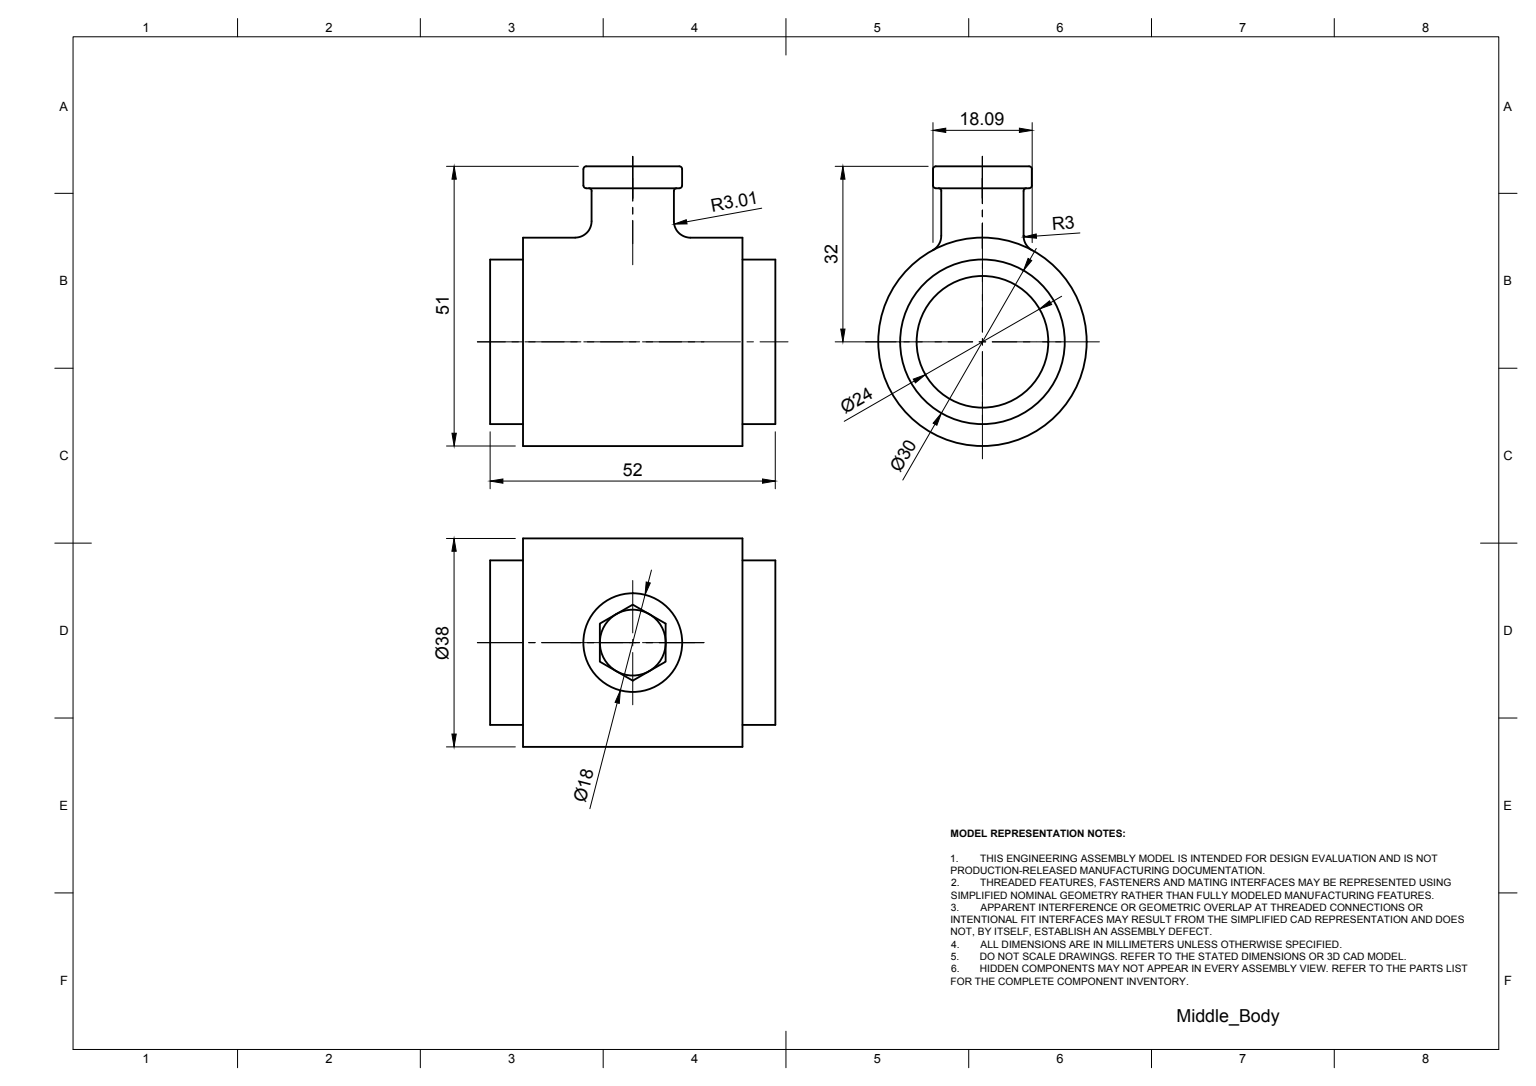
ISO-10303-21;
HEADER;
/* Generated by software containing ST-Developer
 * from STEP Tools, Inc. (www.steptools.com) 
 */

FILE_DESCRIPTION(
/* description */ (''),
/* implementation_level */ '2;1');

FILE_NAME(
/* name */ 'Middle_Body.step',
/* time_stamp */ '2026-10-06T12:47:13-07:00',
/* author */ (''),
/* organization */ (''),
/* preprocessor_version */ 'ST-DEVELOPER v20.2',
/* originating_system */ 'Autodesk Translation Framework v15.15.0.0',
/* authorisation */ '');

FILE_SCHEMA (('AUTOMOTIVE_DESIGN { 1 0 10303 214 3 1 1 }'));
ENDSEC;

DATA;
#10=MECHANICAL_DESIGN_GEOMETRIC_PRESENTATION_REPRESENTATION('',(#67),#42667);
#49=SHAPE_REPRESENTATION_RELATIONSHIP('SRR','None',#42702,#58);
#58=ADVANCED_BREP_SHAPE_REPRESENTATION('',(#76),#42658);
#67=STYLED_ITEM('',(#42756),#76);
#76=MANIFOLD_SOLID_BREP('Body1',#4032);
#85=B_SPLINE_SURFACE_WITH_KNOTS('',3,3,((#5678,#5679,#5680,#5681,#5682,
#5683,#5684,#5685,#5686,#5687,#5688,#5689,#5690,#5691,#5692,#5693,#5694,
#5695),(#5696,#5697,#5698,#5699,#5700,#5701,#5702,#5703,#5704,#5705,#5706,
#5707,#5708,#5709,#5710,#5711,#5712,#5713),(#5714,#5715,#5716,#5717,#5718,
#5719,#5720,#5721,#5722,#5723,#5724,#5725,#5726,#5727,#5728,#5729,#5730,
#5731),(#5732,#5733,#5734,#5735,#5736,#5737,#5738,#5739,#5740,#5741,#5742,
#5743,#5744,#5745,#5746,#5747,#5748,#5749),(#5750,#5751,#5752,#5753,#5754,
#5755,#5756,#5757,#5758,#5759,#5760,#5761,#5762,#5763,#5764,#5765,#5766,
#5767)),.UNSPECIFIED.,.F.,.T.,.F.,(4,1,4),(4,1,1,1,1,1,1,1,1,1,1,1,1,1,
1,4),(0.,0.571428571428571,1.00004196138552),(0.,0.326770108848208,0.653540217696416,
0.980310326544624,1.30708043539283,1.52492717462497,1.96062065308925,2.17846739232139,
2.39631413155352,2.61416087078566,3.04985434924994,3.26770108848208,3.48554782771422,
3.92124130617849,4.2480114150267,4.57478152387491),.UNSPECIFIED.);
#94=B_SPLINE_CURVE_WITH_KNOTS('',3,(#5427,#5428,#5429,#5430,#5431,#5432,
#5433,#5434,#5435,#5436,#5437,#5438,#5439,#5440,#5441,#5442,#5443,#5444,
#5445,#5446,#5447,#5448,#5449,#5450,#5451,#5452,#5453,#5454,#5455,#5456,
#5457,#5458,#5459,#5460,#5461,#5462,#5463,#5464,#5465,#5466,#5467,#5468,
#5469,#5470,#5471,#5472,#5473,#5474,#5475,#5476,#5477,#5478,#5479,#5480,
#5481,#5482,#5483,#5484,#5485,#5486,#5487,#5488,#5489,#5490,#5491,#5492,
#5493,#5494,#5495,#5496,#5497,#5498,#5499,#5500,#5501,#5502,#5503,#5504,
#5505,#5506,#5507,#5508,#5509,#5510,#5511,#5512,#5513,#5514,#5515,#5516,
#5517,#5518,#5519,#5520,#5521,#5522,#5523,#5524,#5525,#5526,#5527,#5528,
#5529,#5530,#5531,#5532,#5533,#5534,#5535,#5536,#5537,#5538,#5539,#5540,
#5541,#5542,#5543,#5544,#5545,#5546,#5547,#5548,#5549,#5550),
 .UNSPECIFIED.,.F.,.F.,(4,3,3,3,3,3,3,3,3,3,3,3,3,3,3,3,3,3,3,3,3,3,3,3,
3,3,3,3,3,3,3,3,3,3,3,3,3,3,3,3,3,4),(0.,0.0515890274929282,0.103204292695659,
0.154856373216778,0.206591856648151,0.25837614825577,0.310254566416546,
0.326770108848208,0.398899776939704,0.480730369472977,0.567135293584696,
0.646990791668246,0.653540217696416,0.713270639311335,0.772778129234328,
0.831949962874738,0.890922354735589,0.949595703830974,0.980310326544624,
1.02811421917601,1.07588590458137,1.1236371825647,1.17139353825776,1.21915060551796,
1.26694469505578,1.30708043539283,1.36339088247901,1.4198291936612,1.47649599617247,
1.52492717462497,1.60478198943241,1.69630632876662,1.79926962978145,1.88030337649094,
1.96062065308925,2.01516322116673,2.0696000908893,2.12403374160535,2.17846739232139,
2.22502234109762,2.27155796869371,2.28737840760206),.UNSPECIFIED.);
#95=B_SPLINE_CURVE_WITH_KNOTS('',3,(#5551,#5552,#5553,#5554,#5555,#5556,
#5557,#5558,#5559,#5560,#5561,#5562,#5563,#5564,#5565,#5566,#5567,#5568,
#5569,#5570,#5571,#5572,#5573,#5574,#5575,#5576,#5577,#5578,#5579,#5580,
#5581,#5582,#5583,#5584,#5585,#5586,#5587,#5588,#5589,#5590,#5591,#5592,
#5593,#5594,#5595,#5596,#5597,#5598,#5599,#5600,#5601,#5602,#5603,#5604,
#5605,#5606,#5607,#5608,#5609,#5610,#5611,#5612,#5613,#5614,#5615,#5616,
#5617,#5618,#5619,#5620,#5621,#5622,#5623,#5624,#5625,#5626,#5627,#5628,
#5629,#5630,#5631,#5632,#5633,#5634,#5635,#5636,#5637,#5638,#5639,#5640,
#5641,#5642,#5643,#5644,#5645,#5646,#5647,#5648,#5649,#5650,#5651,#5652,
#5653,#5654,#5655,#5656,#5657,#5658,#5659,#5660,#5661,#5662,#5663,#5664,
#5665,#5666,#5667,#5668,#5669,#5670,#5671,#5672,#5673,#5674,#5675,#5676,
#5677),.UNSPECIFIED.,.F.,.F.,(4,3,3,3,3,3,3,3,3,3,3,3,3,3,3,3,3,3,3,3,3,
3,3,3,3,3,3,3,3,3,3,3,3,3,3,3,3,3,3,3,3,3,4),(2.28737840766402,2.33375007519743,
2.3801437049756,2.39631413155352,2.45117314344955,2.50612653591306,2.56126498980737,
2.61416087078566,2.69133411582037,2.77539876579215,2.86930017643718,2.95957726284356,
3.0384899988861,3.04985434924994,3.11071114418125,3.17119439820841,3.23109353713712,
3.26770108848208,3.31260298810012,3.35748093451019,3.40234653816875,3.44723256342706,
3.48554782771422,3.54204675587125,3.59866131344456,3.65539681169898,3.712258631246,
3.76933145073308,3.82652040574213,3.8839071682845,3.92124130617849,4.00407786973751,
4.08802290404028,4.16801715953349,4.23929616483205,4.2480114150267,4.30052474757075,
4.35295604051741,4.40531606758536,4.45759990073163,4.50983970731316,4.56203893311869,
4.57478152387491),.UNSPECIFIED.);
#96=B_SPLINE_CURVE_WITH_KNOTS('',3,(#5769,#5770,#5771,#5772,#5773),
 .UNSPECIFIED.,.F.,.F.,(4,1,4),(0.,0.571428571428571,1.00000000000031),
 .UNSPECIFIED.);
#97=B_SPLINE_CURVE_WITH_KNOTS('',3,(#5774,#5775,#5776,#5777,#5778,#5779,
#5780,#5781,#5782,#5783,#5784,#5785,#5786,#5787,#5788,#5789,#5790,#5791),
 .UNSPECIFIED.,.T.,.F.,(4,1,1,1,1,1,1,1,1,1,1,1,1,1,1,4),(-4.57478152387491,
-4.2480114150267,-3.92124130617849,-3.48554782771422,-3.26770108848208,
-3.04985434924994,-2.61416087078566,-2.39631413155352,-2.17846739232139,
-1.96062065308925,-1.52492717462497,-1.30708043539283,-0.980310326544624,
-0.653540217696416,-0.326770108848208,0.),.UNSPECIFIED.);
#98=B_SPLINE_CURVE_WITH_KNOTS('',3,(#5801,#5802,#5803,#5804,#5805,#5806,
#5807,#5808,#5809,#5810,#5811,#5812,#5813,#5814,#5815,#5816,#5817,#5818),
 .UNSPECIFIED.,.F.,.F.,(4,2,2,2,2,2,2,2,4),(-3.69014930019619,-3.45920017966731,
-3.22825105913842,-2.99793151714278,-2.76761197514714,-2.5372924331515,
-2.30697289115586,-2.07602377062698,-1.8450746500981),.UNSPECIFIED.);
#99=B_SPLINE_CURVE_WITH_KNOTS('',3,(#5819,#5820,#5821,#5822,#5823,#5824,
#5825,#5826,#5827,#5828,#5829,#5830,#5831,#5832,#5833,#5834,#5835,#5836),
 .UNSPECIFIED.,.F.,.F.,(4,2,2,2,2,2,2,2,4),(-1.8450746500981,-1.61412552956921,
-1.38317640904033,-1.15285686704469,-0.922537325049048,-0.692217783053408,
-0.461898241057768,-0.230949120528884,0.),.UNSPECIFIED.);
#379=FACE_BOUND('',#851,.T.);
#380=FACE_BOUND('',#854,.T.);
#381=FACE_BOUND('',#859,.T.);
#382=FACE_BOUND('',#863,.T.);
#383=FACE_BOUND('',#866,.T.);
#384=FACE_BOUND('',#868,.T.);
#385=FACE_BOUND('',#870,.T.);
#386=FACE_BOUND('',#872,.T.);
#396=CYLINDRICAL_SURFACE('',#4166,9.);
#397=CYLINDRICAL_SURFACE('',#4178,7.5);
#398=CYLINDRICAL_SURFACE('',#4179,19.);
#399=CYLINDRICAL_SURFACE('',#4182,6.);
#400=CYLINDRICAL_SURFACE('',#4183,15.);
#401=CYLINDRICAL_SURFACE('',#4188,15.);
#402=CYLINDRICAL_SURFACE('',#4193,12.);
#500=TOROIDAL_SURFACE('',#4162,8.5,0.5);
#501=TOROIDAL_SURFACE('',#4169,8.5,0.5);
#502=TOROIDAL_SURFACE('',#4174,8.,0.5);
#519=CIRCLE('',#4148,6.);
#520=CIRCLE('',#4150,6.);
#521=CIRCLE('',#4152,6.);
#522=CIRCLE('',#4154,6.);
#523=CIRCLE('',#4156,6.);
#524=CIRCLE('',#4158,6.);
#525=CIRCLE('',#4159,6.);
#526=CIRCLE('',#4163,8.5);
#527=CIRCLE('',#4164,0.5);
#528=CIRCLE('',#4165,9.);
#529=CIRCLE('',#4167,9.);
#530=CIRCLE('',#4170,0.5);
#531=CIRCLE('',#4171,8.5);
#532=CIRCLE('',#4173,8.);
#533=CIRCLE('',#4175,7.5);
#534=CIRCLE('',#4176,0.5);
#535=CIRCLE('',#4177,7.5);
#536=CIRCLE('',#4180,19.);
#537=CIRCLE('',#4181,19.);
#538=CIRCLE('',#4184,15.);
#539=CIRCLE('',#4185,15.);
#540=CIRCLE('',#4187,12.);
#541=CIRCLE('',#4189,15.);
#542=CIRCLE('',#4190,15.);
#543=CIRCLE('',#4192,12.);
#638=FACE_OUTER_BOUND('',#836,.T.);
#639=FACE_OUTER_BOUND('',#837,.T.);
#640=FACE_OUTER_BOUND('',#838,.T.);
#641=FACE_OUTER_BOUND('',#839,.T.);
#642=FACE_OUTER_BOUND('',#840,.T.);
#643=FACE_OUTER_BOUND('',#841,.T.);
#644=FACE_OUTER_BOUND('',#842,.T.);
#645=FACE_OUTER_BOUND('',#843,.T.);
#646=FACE_OUTER_BOUND('',#844,.T.);
#647=FACE_OUTER_BOUND('',#845,.T.);
#648=FACE_OUTER_BOUND('',#846,.T.);
#649=FACE_OUTER_BOUND('',#847,.T.);
#650=FACE_OUTER_BOUND('',#848,.T.);
#651=FACE_OUTER_BOUND('',#849,.T.);
#652=FACE_OUTER_BOUND('',#850,.T.);
#653=FACE_OUTER_BOUND('',#852,.T.);
#654=FACE_OUTER_BOUND('',#853,.T.);
#655=FACE_OUTER_BOUND('',#855,.T.);
#656=FACE_OUTER_BOUND('',#856,.T.);
#657=FACE_OUTER_BOUND('',#857,.T.);
#658=FACE_OUTER_BOUND('',#858,.T.);
#659=FACE_OUTER_BOUND('',#860,.T.);
#660=FACE_OUTER_BOUND('',#861,.T.);
#661=FACE_OUTER_BOUND('',#862,.T.);
#662=FACE_OUTER_BOUND('',#864,.T.);
#663=FACE_OUTER_BOUND('',#865,.T.);
#664=FACE_OUTER_BOUND('',#867,.T.);
#665=FACE_OUTER_BOUND('',#869,.T.);
#666=FACE_OUTER_BOUND('',#871,.T.);
#836=EDGE_LOOP('',(#2536,#2537,#2538,#2539,#2540));
#837=EDGE_LOOP('',(#2541,#2542,#2543,#2544,#2545));
#838=EDGE_LOOP('',(#2546,#2547,#2548,#2549,#2550));
#839=EDGE_LOOP('',(#2551,#2552,#2553,#2554,#2555));
#840=EDGE_LOOP('',(#2556,#2557,#2558));
#841=EDGE_LOOP('',(#2559,#2560,#2561));
#842=EDGE_LOOP('',(#2562,#2563,#2564));
#843=EDGE_LOOP('',(#2565,#2566,#2567));
#844=EDGE_LOOP('',(#2568,#2569,#2570));
#845=EDGE_LOOP('',(#2571,#2572,#2573,#2574));
#846=EDGE_LOOP('',(#2575,#2576,#2577,#2578,#2579));
#847=EDGE_LOOP('',(#2580,#2581,#2582,#2583,#2584));
#848=EDGE_LOOP('',(#2585,#2586,#2587,#2588));
#849=EDGE_LOOP('',(#2589,#2590,#2591,#2592));
#850=EDGE_LOOP('',(#2593));
#851=EDGE_LOOP('',(#2594,#2595,#2596,#2597,#2598,#2599));
#852=EDGE_LOOP('',(#2600,#2601,#2602,#2603));
#853=EDGE_LOOP('',(#2604));
#854=EDGE_LOOP('',(#2605));
#855=EDGE_LOOP('',(#2606,#2607,#2608,#2609,#2610));
#856=EDGE_LOOP('',(#2611,#2612,#2613,#2614,#2615,#2616));
#857=EDGE_LOOP('',(#2617,#2618,#2619,#2620,#2621));
#858=EDGE_LOOP('',(#2622,#2623,#2624,#2625));
#859=EDGE_LOOP('',(#2626));
#860=EDGE_LOOP('',(#2627,#2628,#2629,#2630,#2631,#2632,#2633,#2634,#2635,
#2636,#2637));
#861=EDGE_LOOP('',(#2638,#2639,#2640,#2641));
#862=EDGE_LOOP('',(#2642));
#863=EDGE_LOOP('',(#2643));
#864=EDGE_LOOP('',(#2644,#2645,#2646,#2647));
#865=EDGE_LOOP('',(#2648));
#866=EDGE_LOOP('',(#2649));
#867=EDGE_LOOP('',(#2650,#2651,#2652,#2653));
#868=EDGE_LOOP('',(#2654,#2655));
#869=EDGE_LOOP('',(#2656));
#870=EDGE_LOOP('',(#2657));
#871=EDGE_LOOP('',(#2658));
#872=EDGE_LOOP('',(#2659));
#1051=LINE('',#5340,#1264);
#1052=LINE('',#5342,#1265);
#1053=LINE('',#5344,#1266);
#1054=LINE('',#5346,#1267);
#1055=LINE('',#5347,#1268);
#1056=LINE('',#5350,#1269);
#1057=LINE('',#5352,#1270);
#1058=LINE('',#5354,#1271);
#1059=LINE('',#5355,#1272);
#1060=LINE('',#5358,#1273);
#1061=LINE('',#5360,#1274);
#1062=LINE('',#5362,#1275);
#1063=LINE('',#5363,#1276);
#1064=LINE('',#5366,#1277);
#1065=LINE('',#5368,#1278);
#1066=LINE('',#5370,#1279);
#1067=LINE('',#5371,#1280);
#1068=LINE('',#5377,#1281);
#1069=LINE('',#5378,#1282);
#1070=LINE('',#5381,#1283);
#1071=LINE('',#5391,#1284);
#1072=LINE('',#5395,#1285);
#1073=LINE('',#5396,#1286);
#1074=LINE('',#5398,#1287);
#1075=LINE('',#5407,#1288);
#1076=LINE('',#5425,#1289);
#1077=LINE('',#5796,#1290);
#1078=LINE('',#5837,#1291);
#1079=LINE('',#5842,#1292);
#1080=LINE('',#5851,#1293);
#1081=LINE('',#5857,#1294);
#1264=VECTOR('',#4474,10.);
#1265=VECTOR('',#4475,10.);
#1266=VECTOR('',#4476,10.);
#1267=VECTOR('',#4477,10.);
#1268=VECTOR('',#4478,10.);
#1269=VECTOR('',#4481,10.);
#1270=VECTOR('',#4482,10.);
#1271=VECTOR('',#4483,10.);
#1272=VECTOR('',#4484,10.);
#1273=VECTOR('',#4487,10.);
#1274=VECTOR('',#4488,10.);
#1275=VECTOR('',#4489,10.);
#1276=VECTOR('',#4490,10.);
#1277=VECTOR('',#4493,9.99999999999999);
#1278=VECTOR('',#4494,10.);
#1279=VECTOR('',#4495,9.99999999999999);
#1280=VECTOR('',#4496,9.99999999999999);
#1281=VECTOR('',#4501,10.);
#1282=VECTOR('',#4502,10.);
#1283=VECTOR('',#4507,10.);
#1284=VECTOR('',#4524,10.);
#1285=VECTOR('',#4529,10.);
#1286=VECTOR('',#4530,10.);
#1287=VECTOR('',#4533,10.);
#1288=VECTOR('',#4544,9.);
#1289=VECTOR('',#4569,7.5);
#1290=VECTOR('',#4574,19.);
#1291=VECTOR('',#4579,6.);
#1292=VECTOR('',#4584,15.);
#1293=VECTOR('',#4595,15.);
#1294=VECTOR('',#4604,12.);
#1477=VERTEX_POINT('',#5338);
#1478=VERTEX_POINT('',#5339);
#1479=VERTEX_POINT('',#5341);
#1480=VERTEX_POINT('',#5343);
#1481=VERTEX_POINT('',#5345);
#1482=VERTEX_POINT('',#5349);
#1483=VERTEX_POINT('',#5351);
#1484=VERTEX_POINT('',#5353);
#1485=VERTEX_POINT('',#5357);
#1486=VERTEX_POINT('',#5359);
#1487=VERTEX_POINT('',#5361);
#1488=VERTEX_POINT('',#5365);
#1489=VERTEX_POINT('',#5367);
#1490=VERTEX_POINT('',#5369);
#1491=VERTEX_POINT('',#5373);
#1492=VERTEX_POINT('',#5374);
#1493=VERTEX_POINT('',#5376);
#1494=VERTEX_POINT('',#5389);
#1495=VERTEX_POINT('',#5394);
#1496=VERTEX_POINT('',#5400);
#1497=VERTEX_POINT('',#5402);
#1498=VERTEX_POINT('',#5406);
#1499=VERTEX_POINT('',#5411);
#1500=VERTEX_POINT('',#5415);
#1501=VERTEX_POINT('',#5418);
#1502=VERTEX_POINT('',#5419);
#1503=VERTEX_POINT('',#5424);
#1504=VERTEX_POINT('',#5426);
#1505=VERTEX_POINT('',#5768);
#1506=VERTEX_POINT('',#5793);
#1507=VERTEX_POINT('',#5795);
#1508=VERTEX_POINT('',#5799);
#1509=VERTEX_POINT('',#5800);
#1510=VERTEX_POINT('',#5839);
#1511=VERTEX_POINT('',#5841);
#1512=VERTEX_POINT('',#5845);
#1513=VERTEX_POINT('',#5848);
#1514=VERTEX_POINT('',#5850);
#1515=VERTEX_POINT('',#5854);
#1919=EDGE_CURVE('',#1477,#1478,#1051,.T.);
#1920=EDGE_CURVE('',#1479,#1477,#1052,.T.);
#1921=EDGE_CURVE('',#1479,#1480,#1053,.T.);
#1922=EDGE_CURVE('',#1480,#1481,#1054,.T.);
#1923=EDGE_CURVE('',#1481,#1478,#1055,.T.);
#1924=EDGE_CURVE('',#1482,#1477,#1056,.T.);
#1925=EDGE_CURVE('',#1483,#1482,#1057,.T.);
#1926=EDGE_CURVE('',#1483,#1484,#1058,.T.);
#1927=EDGE_CURVE('',#1484,#1479,#1059,.T.);
#1928=EDGE_CURVE('',#1478,#1485,#1060,.T.);
#1929=EDGE_CURVE('',#1481,#1486,#1061,.T.);
#1930=EDGE_CURVE('',#1486,#1487,#1062,.T.);
#1931=EDGE_CURVE('',#1487,#1485,#1063,.T.);
#1932=EDGE_CURVE('',#1488,#1482,#1064,.T.);
#1933=EDGE_CURVE('',#1489,#1488,#1065,.T.);
#1934=EDGE_CURVE('',#1489,#1490,#1066,.T.);
#1935=EDGE_CURVE('',#1490,#1483,#1067,.T.);
#1936=EDGE_CURVE('',#1491,#1492,#519,.T.);
#1937=EDGE_CURVE('',#1493,#1491,#1068,.T.);
#1938=EDGE_CURVE('',#1492,#1493,#1069,.T.);
#1939=EDGE_CURVE('',#1492,#1486,#520,.T.);
#1940=EDGE_CURVE('',#1487,#1492,#1070,.T.);
#1941=EDGE_CURVE('',#1486,#1480,#521,.T.);
#1942=EDGE_CURVE('',#1480,#1484,#522,.T.);
#1943=EDGE_CURVE('',#1484,#1490,#523,.T.);
#1944=EDGE_CURVE('',#1490,#1494,#524,.T.);
#1945=EDGE_CURVE('',#1491,#1489,#1071,.T.);
#1946=EDGE_CURVE('',#1494,#1491,#525,.T.);
#1947=EDGE_CURVE('',#1485,#1495,#1072,.T.);
#1948=EDGE_CURVE('',#1495,#1493,#1073,.T.);
#1949=EDGE_CURVE('',#1495,#1488,#1074,.T.);
#1950=EDGE_CURVE('',#1496,#1496,#526,.T.);
#1951=EDGE_CURVE('',#1496,#1497,#527,.T.);
#1952=EDGE_CURVE('',#1497,#1497,#528,.T.);
#1953=EDGE_CURVE('',#1497,#1498,#1075,.T.);
#1954=EDGE_CURVE('',#1498,#1498,#529,.T.);
#1955=EDGE_CURVE('',#1498,#1499,#530,.T.);
#1956=EDGE_CURVE('',#1499,#1499,#531,.T.);
#1957=EDGE_CURVE('',#1500,#1500,#532,.T.);
#1958=EDGE_CURVE('',#1501,#1502,#533,.T.);
#1959=EDGE_CURVE('',#1502,#1500,#534,.T.);
#1960=EDGE_CURVE('',#1502,#1501,#535,.T.);
#1961=EDGE_CURVE('',#1501,#1503,#1076,.T.);
#1962=EDGE_CURVE('',#1504,#1503,#94,.T.);
#1963=EDGE_CURVE('',#1503,#1504,#95,.T.);
#1964=EDGE_CURVE('',#1505,#1504,#96,.T.);
#1965=EDGE_CURVE('',#1505,#1505,#97,.T.);
#1966=EDGE_CURVE('',#1506,#1506,#536,.T.);
#1967=EDGE_CURVE('',#1506,#1507,#1077,.T.);
#1968=EDGE_CURVE('',#1507,#1507,#537,.T.);
#1969=EDGE_CURVE('',#1508,#1509,#98,.T.);
#1970=EDGE_CURVE('',#1509,#1508,#99,.T.);
#1971=EDGE_CURVE('',#1509,#1494,#1078,.T.);
#1972=EDGE_CURVE('',#1510,#1510,#538,.T.);
#1973=EDGE_CURVE('',#1510,#1511,#1079,.T.);
#1974=EDGE_CURVE('',#1511,#1511,#539,.T.);
#1975=EDGE_CURVE('',#1512,#1512,#540,.T.);
#1976=EDGE_CURVE('',#1513,#1513,#541,.T.);
#1977=EDGE_CURVE('',#1513,#1514,#1080,.T.);
#1978=EDGE_CURVE('',#1514,#1514,#542,.T.);
#1979=EDGE_CURVE('',#1515,#1515,#543,.T.);
#1980=EDGE_CURVE('',#1515,#1512,#1081,.T.);
#2536=ORIENTED_EDGE('',*,*,#1919,.F.);
#2537=ORIENTED_EDGE('',*,*,#1920,.F.);
#2538=ORIENTED_EDGE('',*,*,#1921,.T.);
#2539=ORIENTED_EDGE('',*,*,#1922,.T.);
#2540=ORIENTED_EDGE('',*,*,#1923,.T.);
#2541=ORIENTED_EDGE('',*,*,#1924,.F.);
#2542=ORIENTED_EDGE('',*,*,#1925,.F.);
#2543=ORIENTED_EDGE('',*,*,#1926,.T.);
#2544=ORIENTED_EDGE('',*,*,#1927,.T.);
#2545=ORIENTED_EDGE('',*,*,#1920,.T.);
#2546=ORIENTED_EDGE('',*,*,#1928,.F.);
#2547=ORIENTED_EDGE('',*,*,#1923,.F.);
#2548=ORIENTED_EDGE('',*,*,#1929,.T.);
#2549=ORIENTED_EDGE('',*,*,#1930,.T.);
#2550=ORIENTED_EDGE('',*,*,#1931,.T.);
#2551=ORIENTED_EDGE('',*,*,#1932,.F.);
#2552=ORIENTED_EDGE('',*,*,#1933,.F.);
#2553=ORIENTED_EDGE('',*,*,#1934,.T.);
#2554=ORIENTED_EDGE('',*,*,#1935,.T.);
#2555=ORIENTED_EDGE('',*,*,#1925,.T.);
#2556=ORIENTED_EDGE('',*,*,#1936,.F.);
#2557=ORIENTED_EDGE('',*,*,#1937,.F.);
#2558=ORIENTED_EDGE('',*,*,#1938,.F.);
#2559=ORIENTED_EDGE('',*,*,#1939,.F.);
#2560=ORIENTED_EDGE('',*,*,#1940,.F.);
#2561=ORIENTED_EDGE('',*,*,#1930,.F.);
#2562=ORIENTED_EDGE('',*,*,#1941,.F.);
#2563=ORIENTED_EDGE('',*,*,#1929,.F.);
#2564=ORIENTED_EDGE('',*,*,#1922,.F.);
#2565=ORIENTED_EDGE('',*,*,#1942,.F.);
#2566=ORIENTED_EDGE('',*,*,#1921,.F.);
#2567=ORIENTED_EDGE('',*,*,#1927,.F.);
#2568=ORIENTED_EDGE('',*,*,#1943,.F.);
#2569=ORIENTED_EDGE('',*,*,#1926,.F.);
#2570=ORIENTED_EDGE('',*,*,#1935,.F.);
#2571=ORIENTED_EDGE('',*,*,#1944,.F.);
#2572=ORIENTED_EDGE('',*,*,#1934,.F.);
#2573=ORIENTED_EDGE('',*,*,#1945,.F.);
#2574=ORIENTED_EDGE('',*,*,#1946,.F.);
#2575=ORIENTED_EDGE('',*,*,#1947,.F.);
#2576=ORIENTED_EDGE('',*,*,#1931,.F.);
#2577=ORIENTED_EDGE('',*,*,#1940,.T.);
#2578=ORIENTED_EDGE('',*,*,#1938,.T.);
#2579=ORIENTED_EDGE('',*,*,#1948,.F.);
#2580=ORIENTED_EDGE('',*,*,#1949,.F.);
#2581=ORIENTED_EDGE('',*,*,#1948,.T.);
#2582=ORIENTED_EDGE('',*,*,#1937,.T.);
#2583=ORIENTED_EDGE('',*,*,#1945,.T.);
#2584=ORIENTED_EDGE('',*,*,#1933,.T.);
#2585=ORIENTED_EDGE('',*,*,#1950,.T.);
#2586=ORIENTED_EDGE('',*,*,#1951,.T.);
#2587=ORIENTED_EDGE('',*,*,#1952,.T.);
#2588=ORIENTED_EDGE('',*,*,#1951,.F.);
#2589=ORIENTED_EDGE('',*,*,#1952,.F.);
#2590=ORIENTED_EDGE('',*,*,#1953,.T.);
#2591=ORIENTED_EDGE('',*,*,#1954,.F.);
#2592=ORIENTED_EDGE('',*,*,#1953,.F.);
#2593=ORIENTED_EDGE('',*,*,#1950,.F.);
#2594=ORIENTED_EDGE('',*,*,#1949,.T.);
#2595=ORIENTED_EDGE('',*,*,#1932,.T.);
#2596=ORIENTED_EDGE('',*,*,#1924,.T.);
#2597=ORIENTED_EDGE('',*,*,#1919,.T.);
#2598=ORIENTED_EDGE('',*,*,#1928,.T.);
#2599=ORIENTED_EDGE('',*,*,#1947,.T.);
#2600=ORIENTED_EDGE('',*,*,#1954,.T.);
#2601=ORIENTED_EDGE('',*,*,#1955,.T.);
#2602=ORIENTED_EDGE('',*,*,#1956,.T.);
#2603=ORIENTED_EDGE('',*,*,#1955,.F.);
#2604=ORIENTED_EDGE('',*,*,#1956,.F.);
#2605=ORIENTED_EDGE('',*,*,#1957,.F.);
#2606=ORIENTED_EDGE('',*,*,#1958,.T.);
#2607=ORIENTED_EDGE('',*,*,#1959,.T.);
#2608=ORIENTED_EDGE('',*,*,#1957,.T.);
#2609=ORIENTED_EDGE('',*,*,#1959,.F.);
#2610=ORIENTED_EDGE('',*,*,#1960,.T.);
#2611=ORIENTED_EDGE('',*,*,#1958,.F.);
#2612=ORIENTED_EDGE('',*,*,#1961,.T.);
#2613=ORIENTED_EDGE('',*,*,#1962,.F.);
#2614=ORIENTED_EDGE('',*,*,#1963,.F.);
#2615=ORIENTED_EDGE('',*,*,#1961,.F.);
#2616=ORIENTED_EDGE('',*,*,#1960,.F.);
#2617=ORIENTED_EDGE('',*,*,#1964,.T.);
#2618=ORIENTED_EDGE('',*,*,#1962,.T.);
#2619=ORIENTED_EDGE('',*,*,#1963,.T.);
#2620=ORIENTED_EDGE('',*,*,#1964,.F.);
#2621=ORIENTED_EDGE('',*,*,#1965,.T.);
#2622=ORIENTED_EDGE('',*,*,#1966,.F.);
#2623=ORIENTED_EDGE('',*,*,#1967,.T.);
#2624=ORIENTED_EDGE('',*,*,#1968,.F.);
#2625=ORIENTED_EDGE('',*,*,#1967,.F.);
#2626=ORIENTED_EDGE('',*,*,#1965,.F.);
#2627=ORIENTED_EDGE('',*,*,#1969,.F.);
#2628=ORIENTED_EDGE('',*,*,#1970,.F.);
#2629=ORIENTED_EDGE('',*,*,#1971,.T.);
#2630=ORIENTED_EDGE('',*,*,#1946,.T.);
#2631=ORIENTED_EDGE('',*,*,#1936,.T.);
#2632=ORIENTED_EDGE('',*,*,#1939,.T.);
#2633=ORIENTED_EDGE('',*,*,#1941,.T.);
#2634=ORIENTED_EDGE('',*,*,#1942,.T.);
#2635=ORIENTED_EDGE('',*,*,#1943,.T.);
#2636=ORIENTED_EDGE('',*,*,#1944,.T.);
#2637=ORIENTED_EDGE('',*,*,#1971,.F.);
#2638=ORIENTED_EDGE('',*,*,#1972,.F.);
#2639=ORIENTED_EDGE('',*,*,#1973,.T.);
#2640=ORIENTED_EDGE('',*,*,#1974,.T.);
#2641=ORIENTED_EDGE('',*,*,#1973,.F.);
#2642=ORIENTED_EDGE('',*,*,#1974,.F.);
#2643=ORIENTED_EDGE('',*,*,#1975,.F.);
#2644=ORIENTED_EDGE('',*,*,#1976,.F.);
#2645=ORIENTED_EDGE('',*,*,#1977,.T.);
#2646=ORIENTED_EDGE('',*,*,#1978,.F.);
#2647=ORIENTED_EDGE('',*,*,#1977,.F.);
#2648=ORIENTED_EDGE('',*,*,#1976,.T.);
#2649=ORIENTED_EDGE('',*,*,#1979,.T.);
#2650=ORIENTED_EDGE('',*,*,#1979,.F.);
#2651=ORIENTED_EDGE('',*,*,#1980,.T.);
#2652=ORIENTED_EDGE('',*,*,#1975,.T.);
#2653=ORIENTED_EDGE('',*,*,#1980,.F.);
#2654=ORIENTED_EDGE('',*,*,#1969,.T.);
#2655=ORIENTED_EDGE('',*,*,#1970,.T.);
#2656=ORIENTED_EDGE('',*,*,#1968,.T.);
#2657=ORIENTED_EDGE('',*,*,#1978,.T.);
#2658=ORIENTED_EDGE('',*,*,#1966,.T.);
#2659=ORIENTED_EDGE('',*,*,#1972,.T.);
#3770=PLANE('',#4143);
#3771=PLANE('',#4144);
#3772=PLANE('',#4145);
#3773=PLANE('',#4146);
#3774=PLANE('',#4147);
#3775=PLANE('',#4149);
#3776=PLANE('',#4151);
#3777=PLANE('',#4153);
#3778=PLANE('',#4155);
#3779=PLANE('',#4157);
#3780=PLANE('',#4160);
#3781=PLANE('',#4161);
#3782=PLANE('',#4168);
#3783=PLANE('',#4172);
#3784=PLANE('',#4186);
#3785=PLANE('',#4191);
#3786=PLANE('',#4194);
#3787=PLANE('',#4195);
#3834=ADVANCED_FACE('',(#638),#3770,.F.);
#3835=ADVANCED_FACE('',(#639),#3771,.F.);
#3836=ADVANCED_FACE('',(#640),#3772,.F.);
#3837=ADVANCED_FACE('',(#641),#3773,.F.);
#3838=ADVANCED_FACE('',(#642),#3774,.F.);
#3839=ADVANCED_FACE('',(#643),#3775,.F.);
#3840=ADVANCED_FACE('',(#644),#3776,.F.);
#3841=ADVANCED_FACE('',(#645),#3777,.F.);
#3842=ADVANCED_FACE('',(#646),#3778,.F.);
#3843=ADVANCED_FACE('',(#647),#3779,.F.);
#3844=ADVANCED_FACE('',(#648),#3780,.F.);
#3845=ADVANCED_FACE('',(#649),#3781,.F.);
#3846=ADVANCED_FACE('',(#650),#500,.T.);
#3847=ADVANCED_FACE('',(#651),#396,.T.);
#3848=ADVANCED_FACE('',(#652,#379),#3782,.T.);
#3849=ADVANCED_FACE('',(#653),#501,.T.);
#3850=ADVANCED_FACE('',(#654,#380),#3783,.F.);
#3851=ADVANCED_FACE('',(#655),#502,.F.);
#3852=ADVANCED_FACE('',(#656),#397,.T.);
#3853=ADVANCED_FACE('',(#657),#85,.T.);
#3854=ADVANCED_FACE('',(#658,#381),#398,.T.);
#3855=ADVANCED_FACE('',(#659),#399,.F.);
#3856=ADVANCED_FACE('',(#660),#400,.T.);
#3857=ADVANCED_FACE('',(#661,#382),#3784,.F.);
#3858=ADVANCED_FACE('',(#662),#401,.T.);
#3859=ADVANCED_FACE('',(#663,#383),#3785,.T.);
#3860=ADVANCED_FACE('',(#664,#384),#402,.F.);
#3861=ADVANCED_FACE('',(#665,#385),#3786,.F.);
#3862=ADVANCED_FACE('',(#666,#386),#3787,.T.);
#4032=CLOSED_SHELL('',(#3834,#3835,#3836,#3837,#3838,#3839,#3840,#3841,
#3842,#3843,#3844,#3845,#3846,#3847,#3848,#3849,#3850,#3851,#3852,#3853,
#3854,#3855,#3856,#3857,#3858,#3859,#3860,#3861,#3862));
#4142=AXIS2_PLACEMENT_3D('',#5336,#4470,#4471);
#4143=AXIS2_PLACEMENT_3D('',#5337,#4472,#4473);
#4144=AXIS2_PLACEMENT_3D('',#5348,#4479,#4480);
#4145=AXIS2_PLACEMENT_3D('',#5356,#4485,#4486);
#4146=AXIS2_PLACEMENT_3D('',#5364,#4491,#4492);
#4147=AXIS2_PLACEMENT_3D('',#5372,#4497,#4498);
#4148=AXIS2_PLACEMENT_3D('',#5375,#4499,#4500);
#4149=AXIS2_PLACEMENT_3D('',#5379,#4503,#4504);
#4150=AXIS2_PLACEMENT_3D('',#5380,#4505,#4506);
#4151=AXIS2_PLACEMENT_3D('',#5382,#4508,#4509);
#4152=AXIS2_PLACEMENT_3D('',#5383,#4510,#4511);
#4153=AXIS2_PLACEMENT_3D('',#5384,#4512,#4513);
#4154=AXIS2_PLACEMENT_3D('',#5385,#4514,#4515);
#4155=AXIS2_PLACEMENT_3D('',#5386,#4516,#4517);
#4156=AXIS2_PLACEMENT_3D('',#5387,#4518,#4519);
#4157=AXIS2_PLACEMENT_3D('',#5388,#4520,#4521);
#4158=AXIS2_PLACEMENT_3D('',#5390,#4522,#4523);
#4159=AXIS2_PLACEMENT_3D('',#5392,#4525,#4526);
#4160=AXIS2_PLACEMENT_3D('',#5393,#4527,#4528);
#4161=AXIS2_PLACEMENT_3D('',#5397,#4531,#4532);
#4162=AXIS2_PLACEMENT_3D('',#5399,#4534,#4535);
#4163=AXIS2_PLACEMENT_3D('',#5401,#4536,#4537);
#4164=AXIS2_PLACEMENT_3D('',#5403,#4538,#4539);
#4165=AXIS2_PLACEMENT_3D('',#5404,#4540,#4541);
#4166=AXIS2_PLACEMENT_3D('',#5405,#4542,#4543);
#4167=AXIS2_PLACEMENT_3D('',#5408,#4545,#4546);
#4168=AXIS2_PLACEMENT_3D('',#5409,#4547,#4548);
#4169=AXIS2_PLACEMENT_3D('',#5410,#4549,#4550);
#4170=AXIS2_PLACEMENT_3D('',#5412,#4551,#4552);
#4171=AXIS2_PLACEMENT_3D('',#5413,#4553,#4554);
#4172=AXIS2_PLACEMENT_3D('',#5414,#4555,#4556);
#4173=AXIS2_PLACEMENT_3D('',#5416,#4557,#4558);
#4174=AXIS2_PLACEMENT_3D('',#5417,#4559,#4560);
#4175=AXIS2_PLACEMENT_3D('',#5420,#4561,#4562);
#4176=AXIS2_PLACEMENT_3D('',#5421,#4563,#4564);
#4177=AXIS2_PLACEMENT_3D('',#5422,#4565,#4566);
#4178=AXIS2_PLACEMENT_3D('',#5423,#4567,#4568);
#4179=AXIS2_PLACEMENT_3D('',#5792,#4570,#4571);
#4180=AXIS2_PLACEMENT_3D('',#5794,#4572,#4573);
#4181=AXIS2_PLACEMENT_3D('',#5797,#4575,#4576);
#4182=AXIS2_PLACEMENT_3D('',#5798,#4577,#4578);
#4183=AXIS2_PLACEMENT_3D('',#5838,#4580,#4581);
#4184=AXIS2_PLACEMENT_3D('',#5840,#4582,#4583);
#4185=AXIS2_PLACEMENT_3D('',#5843,#4585,#4586);
#4186=AXIS2_PLACEMENT_3D('',#5844,#4587,#4588);
#4187=AXIS2_PLACEMENT_3D('',#5846,#4589,#4590);
#4188=AXIS2_PLACEMENT_3D('',#5847,#4591,#4592);
#4189=AXIS2_PLACEMENT_3D('',#5849,#4593,#4594);
#4190=AXIS2_PLACEMENT_3D('',#5852,#4596,#4597);
#4191=AXIS2_PLACEMENT_3D('',#5853,#4598,#4599);
#4192=AXIS2_PLACEMENT_3D('',#5855,#4600,#4601);
#4193=AXIS2_PLACEMENT_3D('',#5856,#4602,#4603);
#4194=AXIS2_PLACEMENT_3D('',#5858,#4605,#4606);
#4195=AXIS2_PLACEMENT_3D('',#5859,#4607,#4608);
#4470=DIRECTION('axis',(0.,0.,1.));
#4471=DIRECTION('refdir',(1.,0.,0.));
#4472=DIRECTION('center_axis',(0.866025403784439,0.5,0.));
#4473=DIRECTION('ref_axis',(0.5,-0.866025403784439,0.));
#4474=DIRECTION('',(0.5,-0.866025403784439,0.));
#4475=DIRECTION('',(0.,0.,1.));
#4476=DIRECTION('',(0.5,-0.866025403784439,0.));
#4477=DIRECTION('',(0.5,-0.866025403784439,0.));
#4478=DIRECTION('',(0.,0.,1.));
#4479=DIRECTION('center_axis',(3.20493781063927E-16,1.,0.));
#4480=DIRECTION('ref_axis',(1.,-3.20493781063927E-16,0.));
#4481=DIRECTION('',(1.,-3.20493781063927E-16,0.));
#4482=DIRECTION('',(0.,0.,1.));
#4483=DIRECTION('',(1.,-3.20493781063927E-16,0.));
#4484=DIRECTION('',(1.,-3.20493781063927E-16,0.));
#4485=DIRECTION('center_axis',(0.866025403784439,-0.5,0.));
#4486=DIRECTION('ref_axis',(-0.5,-0.866025403784439,0.));
#4487=DIRECTION('',(-0.5,-0.866025403784439,0.));
#4488=DIRECTION('',(-0.5,-0.866025403784439,0.));
#4489=DIRECTION('',(-0.5,-0.866025403784439,0.));
#4490=DIRECTION('',(0.,0.,1.));
#4491=DIRECTION('center_axis',(-0.866025403784438,0.5,0.));
#4492=DIRECTION('ref_axis',(0.5,0.866025403784438,0.));
#4493=DIRECTION('',(0.5,0.866025403784439,0.));
#4494=DIRECTION('',(0.,0.,1.));
#4495=DIRECTION('',(0.5,0.866025403784439,0.));
#4496=DIRECTION('',(0.5,0.866025403784439,0.));
#4497=DIRECTION('center_axis',(0.,0.,-1.));
#4498=DIRECTION('ref_axis',(-1.,0.,0.));
#4499=DIRECTION('center_axis',(0.,0.,1.));
#4500=DIRECTION('ref_axis',(1.,0.,0.));
#4501=DIRECTION('',(-0.499999999999999,0.866025403784439,0.));
#4502=DIRECTION('',(-1.,6.40987562127854E-16,0.));
#4503=DIRECTION('center_axis',(0.,0.,-1.));
#4504=DIRECTION('ref_axis',(-1.,0.,0.));
#4505=DIRECTION('center_axis',(0.,0.,1.));
#4506=DIRECTION('ref_axis',(1.,0.,0.));
#4507=DIRECTION('',(-1.,6.40987562127854E-16,0.));
#4508=DIRECTION('center_axis',(0.,0.,-1.));
#4509=DIRECTION('ref_axis',(-1.,0.,0.));
#4510=DIRECTION('center_axis',(0.,0.,1.));
#4511=DIRECTION('ref_axis',(1.,0.,0.));
#4512=DIRECTION('center_axis',(0.,0.,-1.));
#4513=DIRECTION('ref_axis',(-1.,0.,0.));
#4514=DIRECTION('center_axis',(0.,0.,1.));
#4515=DIRECTION('ref_axis',(1.,0.,0.));
#4516=DIRECTION('center_axis',(0.,0.,-1.));
#4517=DIRECTION('ref_axis',(-1.,0.,0.));
#4518=DIRECTION('center_axis',(0.,0.,1.));
#4519=DIRECTION('ref_axis',(1.,0.,0.));
#4520=DIRECTION('center_axis',(0.,0.,-1.));
#4521=DIRECTION('ref_axis',(-1.,0.,0.));
#4522=DIRECTION('center_axis',(0.,0.,1.));
#4523=DIRECTION('ref_axis',(1.,0.,0.));
#4524=DIRECTION('',(-0.499999999999999,0.866025403784439,0.));
#4525=DIRECTION('center_axis',(0.,0.,1.));
#4526=DIRECTION('ref_axis',(1.,0.,0.));
#4527=DIRECTION('center_axis',(-6.40987562127854E-16,-1.,0.));
#4528=DIRECTION('ref_axis',(-1.,6.40987562127854E-16,0.));
#4529=DIRECTION('',(-1.,6.40987562127854E-16,0.));
#4530=DIRECTION('',(0.,0.,-1.));
#4531=DIRECTION('center_axis',(-0.866025403784439,-0.5,0.));
#4532=DIRECTION('ref_axis',(-0.5,0.866025403784439,0.));
#4533=DIRECTION('',(-0.499999999999999,0.866025403784439,0.));
#4534=DIRECTION('center_axis',(0.,0.,1.));
#4535=DIRECTION('ref_axis',(1.,0.,0.));
#4536=DIRECTION('center_axis',(0.,0.,-1.));
#4537=DIRECTION('ref_axis',(1.,0.,0.));
#4538=DIRECTION('center_axis',(1.22464679914735E-16,-1.,0.));
#4539=DIRECTION('ref_axis',(-1.,-1.22464679914735E-16,0.));
#4540=DIRECTION('center_axis',(0.,0.,1.));
#4541=DIRECTION('ref_axis',(1.,0.,0.));
#4542=DIRECTION('center_axis',(0.,0.,1.));
#4543=DIRECTION('ref_axis',(1.,0.,0.));
#4544=DIRECTION('',(0.,0.,-1.));
#4545=DIRECTION('center_axis',(0.,0.,-1.));
#4546=DIRECTION('ref_axis',(1.,0.,0.));
#4547=DIRECTION('center_axis',(0.,0.,1.));
#4548=DIRECTION('ref_axis',(1.,0.,0.));
#4549=DIRECTION('center_axis',(0.,0.,1.));
#4550=DIRECTION('ref_axis',(1.,0.,0.));
#4551=DIRECTION('center_axis',(1.22464679914735E-16,-1.,0.));
#4552=DIRECTION('ref_axis',(-1.,-1.22464679914735E-16,0.));
#4553=DIRECTION('center_axis',(0.,0.,1.));
#4554=DIRECTION('ref_axis',(1.,0.,0.));
#4555=DIRECTION('center_axis',(0.,0.,1.));
#4556=DIRECTION('ref_axis',(1.,0.,0.));
#4557=DIRECTION('center_axis',(0.,0.,-1.));
#4558=DIRECTION('ref_axis',(1.,0.,0.));
#4559=DIRECTION('center_axis',(0.,0.,-1.));
#4560=DIRECTION('ref_axis',(-1.,0.,0.));
#4561=DIRECTION('center_axis',(0.,0.,1.));
#4562=DIRECTION('ref_axis',(1.,0.,0.));
#4563=DIRECTION('center_axis',(1.22464679914735E-16,1.,0.));
#4564=DIRECTION('ref_axis',(1.,-1.22464679914735E-16,0.));
#4565=DIRECTION('center_axis',(0.,0.,1.));
#4566=DIRECTION('ref_axis',(1.,0.,0.));
#4567=DIRECTION('center_axis',(0.,0.,1.));
#4568=DIRECTION('ref_axis',(1.,0.,0.));
#4569=DIRECTION('',(0.,0.,-1.));
#4570=DIRECTION('center_axis',(0.,1.,0.));
#4571=DIRECTION('ref_axis',(1.,0.,0.));
#4572=DIRECTION('center_axis',(0.,1.,0.));
#4573=DIRECTION('ref_axis',(1.,0.,0.));
#4574=DIRECTION('',(0.,-1.,0.));
#4575=DIRECTION('center_axis',(0.,-1.,0.));
#4576=DIRECTION('ref_axis',(1.,0.,0.));
#4577=DIRECTION('center_axis',(0.,0.,1.));
#4578=DIRECTION('ref_axis',(1.,0.,0.));
#4579=DIRECTION('',(0.,0.,1.));
#4580=DIRECTION('center_axis',(0.,-1.,0.));
#4581=DIRECTION('ref_axis',(1.,0.,0.));
#4582=DIRECTION('center_axis',(0.,-1.,0.));
#4583=DIRECTION('ref_axis',(1.,0.,0.));
#4584=DIRECTION('',(0.,1.,0.));
#4585=DIRECTION('center_axis',(0.,-1.,0.));
#4586=DIRECTION('ref_axis',(1.,0.,0.));
#4587=DIRECTION('center_axis',(0.,-1.,0.));
#4588=DIRECTION('ref_axis',(1.,0.,0.));
#4589=DIRECTION('center_axis',(0.,1.,0.));
#4590=DIRECTION('ref_axis',(1.,0.,0.));
#4591=DIRECTION('center_axis',(0.,-1.,0.));
#4592=DIRECTION('ref_axis',(1.,0.,0.));
#4593=DIRECTION('center_axis',(0.,-1.,0.));
#4594=DIRECTION('ref_axis',(1.,0.,0.));
#4595=DIRECTION('',(0.,1.,0.));
#4596=DIRECTION('center_axis',(0.,1.,0.));
#4597=DIRECTION('ref_axis',(1.,0.,0.));
#4598=DIRECTION('center_axis',(0.,-1.,0.));
#4599=DIRECTION('ref_axis',(1.,0.,0.));
#4600=DIRECTION('center_axis',(0.,1.,0.));
#4601=DIRECTION('ref_axis',(1.,0.,0.));
#4602=DIRECTION('center_axis',(0.,1.,0.));
#4603=DIRECTION('ref_axis',(1.,0.,0.));
#4604=DIRECTION('',(0.,1.,0.));
#4605=DIRECTION('center_axis',(0.,1.,0.));
#4606=DIRECTION('ref_axis',(1.,0.,0.));
#4607=DIRECTION('center_axis',(0.,1.,0.));
#4608=DIRECTION('ref_axis',(1.,0.,0.));
#5336=CARTESIAN_POINT('',(0.,0.,0.));
#5337=CARTESIAN_POINT('Origin',(3.46410161513776,6.,32.));
#5338=CARTESIAN_POINT('',(3.46410161513776,6.,32.));
#5339=CARTESIAN_POINT('',(6.92820323027551,-2.22044604925031E-15,32.));
#5340=CARTESIAN_POINT('',(4.3301270189222,4.5,32.));
#5341=CARTESIAN_POINT('',(3.46410161513776,6.,29.));
#5342=CARTESIAN_POINT('',(3.46410161513776,6.,32.));
#5343=CARTESIAN_POINT('',(5.19615242270663,3.,29.));
#5344=CARTESIAN_POINT('',(6.92820323027551,-2.22044604925031E-15,29.));
#5345=CARTESIAN_POINT('',(6.92820323027551,-2.22044604925031E-15,29.));
#5346=CARTESIAN_POINT('',(6.92820323027551,-2.22044604925031E-15,29.));
#5347=CARTESIAN_POINT('',(6.92820323027551,-2.22044604925031E-15,32.));
#5348=CARTESIAN_POINT('Origin',(-3.46410161513775,6.,32.));
#5349=CARTESIAN_POINT('',(-3.46410161513775,6.,32.));
#5350=CARTESIAN_POINT('',(-1.73205080756887,6.,32.));
#5351=CARTESIAN_POINT('',(-3.46410161513775,6.,29.));
#5352=CARTESIAN_POINT('',(-3.46410161513775,6.,32.));
#5353=CARTESIAN_POINT('',(1.94289029309402E-15,6.,29.));
#5354=CARTESIAN_POINT('',(3.46410161513776,6.,29.));
#5355=CARTESIAN_POINT('',(3.46410161513776,6.,29.));
#5356=CARTESIAN_POINT('Origin',(6.92820323027551,-2.22044604925031E-15,
32.));
#5357=CARTESIAN_POINT('',(3.46410161513775,-6.,32.));
#5358=CARTESIAN_POINT('',(6.06217782649107,-1.5,32.));
#5359=CARTESIAN_POINT('',(5.19615242270663,-3.,29.));
#5360=CARTESIAN_POINT('',(3.46410161513775,-6.,29.));
#5361=CARTESIAN_POINT('',(3.46410161513775,-6.,29.));
#5362=CARTESIAN_POINT('',(3.46410161513775,-6.,29.));
#5363=CARTESIAN_POINT('',(3.46410161513775,-6.,32.));
#5364=CARTESIAN_POINT('Origin',(-6.92820323027551,4.44089209850063E-15,
32.));
#5365=CARTESIAN_POINT('',(-6.92820323027551,3.88578058618805E-15,32.));
#5366=CARTESIAN_POINT('',(-6.06217782649107,1.5,32.));
#5367=CARTESIAN_POINT('',(-6.92820323027551,4.44089209850063E-15,29.));
#5368=CARTESIAN_POINT('',(-6.92820323027551,3.88578058618805E-15,32.));
#5369=CARTESIAN_POINT('',(-5.19615242270663,3.,29.));
#5370=CARTESIAN_POINT('',(-3.46410161513775,6.,29.));
#5371=CARTESIAN_POINT('',(-3.46410161513775,6.,29.));
#5372=CARTESIAN_POINT('Origin',(0.,0.,29.));
#5373=CARTESIAN_POINT('',(-5.19615242270663,-3.,29.));
#5374=CARTESIAN_POINT('',(-3.88578058618805E-15,-6.,29.));
#5375=CARTESIAN_POINT('Origin',(0.,0.,29.));
#5376=CARTESIAN_POINT('',(-3.46410161513776,-6.,29.));
#5377=CARTESIAN_POINT('',(-6.92820323027551,3.88578058618805E-15,29.));
#5378=CARTESIAN_POINT('',(-3.46410161513776,-6.,29.));
#5379=CARTESIAN_POINT('Origin',(0.,0.,29.));
#5380=CARTESIAN_POINT('Origin',(0.,0.,29.));
#5381=CARTESIAN_POINT('',(-3.46410161513776,-6.,29.));
#5382=CARTESIAN_POINT('Origin',(0.,0.,29.));
#5383=CARTESIAN_POINT('Origin',(0.,0.,29.));
#5384=CARTESIAN_POINT('Origin',(0.,0.,29.));
#5385=CARTESIAN_POINT('Origin',(0.,0.,29.));
#5386=CARTESIAN_POINT('Origin',(0.,0.,29.));
#5387=CARTESIAN_POINT('Origin',(0.,0.,29.));
#5388=CARTESIAN_POINT('Origin',(0.,0.,29.));
#5389=CARTESIAN_POINT('',(-6.,-7.34788079488412E-16,29.));
#5390=CARTESIAN_POINT('Origin',(0.,0.,29.));
#5391=CARTESIAN_POINT('',(-6.92820323027551,3.88578058618805E-15,29.));
#5392=CARTESIAN_POINT('Origin',(0.,0.,29.));
#5393=CARTESIAN_POINT('Origin',(3.46410161513775,-6.,32.));
#5394=CARTESIAN_POINT('',(-3.46410161513776,-6.,32.));
#5395=CARTESIAN_POINT('',(1.73205080756887,-6.,32.));
#5396=CARTESIAN_POINT('',(-3.46410161513776,-6.,32.));
#5397=CARTESIAN_POINT('Origin',(-3.46410161513776,-6.,32.));
#5398=CARTESIAN_POINT('',(-4.3301270189222,-4.5,32.));
#5399=CARTESIAN_POINT('Origin',(0.,0.,31.5));
#5400=CARTESIAN_POINT('',(-8.5,1.04094977927525E-15,32.));
#5401=CARTESIAN_POINT('Origin',(0.,0.,32.));
#5402=CARTESIAN_POINT('',(-9.,-1.10218211923262E-15,31.5));
#5403=CARTESIAN_POINT('Origin',(-8.5,-1.04094977927525E-15,31.5));
#5404=CARTESIAN_POINT('Origin',(0.,0.,31.5));
#5405=CARTESIAN_POINT('Origin',(0.,0.,0.));
#5406=CARTESIAN_POINT('',(-9.,1.10218211923262E-15,28.5));
#5407=CARTESIAN_POINT('',(-9.,-1.10218211923262E-15,0.));
#5408=CARTESIAN_POINT('Origin',(0.,0.,28.5));
#5409=CARTESIAN_POINT('Origin',(0.,0.,32.));
#5410=CARTESIAN_POINT('Origin',(0.,0.,28.5));
#5411=CARTESIAN_POINT('',(-8.5,-1.04094977927525E-15,28.));
#5412=CARTESIAN_POINT('Origin',(-8.5,-1.04094977927525E-15,28.5));
#5413=CARTESIAN_POINT('Origin',(0.,0.,28.));
#5414=CARTESIAN_POINT('Origin',(0.,0.,28.));
#5415=CARTESIAN_POINT('',(8.,-9.79717439317883E-16,28.));
#5416=CARTESIAN_POINT('Origin',(0.,0.,28.));
#5417=CARTESIAN_POINT('Origin',(0.,0.,27.5));
#5418=CARTESIAN_POINT('',(-7.5,-9.18485099360515E-16,27.5));
#5419=CARTESIAN_POINT('',(7.5,-9.18485099360515E-16,27.5));
#5420=CARTESIAN_POINT('Origin',(0.,0.,27.5));
#5421=CARTESIAN_POINT('Origin',(8.,-9.79717439317883E-16,27.5));
#5422=CARTESIAN_POINT('Origin',(0.,0.,27.5));
#5423=CARTESIAN_POINT('Origin',(0.,0.,0.));
#5424=CARTESIAN_POINT('',(-7.49999999972844,-6.38227930889562E-5,19.332958859286));
#5425=CARTESIAN_POINT('',(-7.5,-9.18485099360515E-16,0.));
#5426=CARTESIAN_POINT('',(7.5,-2.77555756156289E-16,19.3326149291812));
#5427=CARTESIAN_POINT('Ctrl Pts',(7.5,1.82323373546694E-16,19.3326149291812));
#5428=CARTESIAN_POINT('Ctrl Pts',(7.5,-0.179953506202678,19.3326149291812));
#5429=CARTESIAN_POINT('Ctrl Pts',(7.49351901743291,-0.35981913831206,19.3379986486473));
#5430=CARTESIAN_POINT('Ctrl Pts',(7.48060194606833,-0.539068200210999,19.348331639646));
#5431=CARTESIAN_POINT('Ctrl Pts',(7.46767830519883,-0.718408426551234,19.3586698859099));
#5432=CARTESIAN_POINT('Ctrl Pts',(7.44831209315138,-0.897131076731049,19.3739624392954));
#5433=CARTESIAN_POINT('Ctrl Pts',(7.42259977836276,-1.07471509259388,19.393774188663));
#5434=CARTESIAN_POINT('Ctrl Pts',(7.39686912390173,-1.25242577276927,19.4136000690412));
#5435=CARTESIAN_POINT('Ctrl Pts',(7.36478341945685,-1.42899582546002,19.4379515944617));
#5436=CARTESIAN_POINT('Ctrl Pts',(7.32648959561089,-1.60391714418337,19.466392722073));
#5437=CARTESIAN_POINT('Ctrl Pts',(7.28813393850825,-1.77912090936192,19.494879773736));
#5438=CARTESIAN_POINT('Ctrl Pts',(7.24355024225288,-1.95267025573421,19.5274696452608));
#5439=CARTESIAN_POINT('Ctrl Pts',(7.19293465289676,-2.12407416988132,19.5637241781409));
#5440=CARTESIAN_POINT('Ctrl Pts',(7.1422713118924,-2.29563978953298,19.6000129141928));
#5441=CARTESIAN_POINT('Ctrl Pts',(7.0855648826377,-2.46505559387656,19.6399732294753));
#5442=CARTESIAN_POINT('Ctrl Pts',(7.0230580843623,-2.63185393661452,19.6831657242118));
#5443=CARTESIAN_POINT('Ctrl Pts',(6.96043766959649,-2.79895546305137,19.7264367284834));
#5444=CARTESIAN_POINT('Ctrl Pts',(6.89199600386832,-2.96342969182938,19.7729516729341));
#5445=CARTESIAN_POINT('Ctrl Pts',(6.81802018505874,-3.12483611668381,19.8222687573836));
#5446=CARTESIAN_POINT('Ctrl Pts',(6.79446991468079,-3.17622000140761,19.8379688968579));
#5447=CARTESIAN_POINT('Ctrl Pts',(6.77035908491064,-3.22729321641509,19.8539530256882));
#5448=CARTESIAN_POINT('Ctrl Pts',(6.74569781201533,-3.27804225551953,19.8702068896288));
#5449=CARTESIAN_POINT('Ctrl Pts',(6.63799263454312,-3.49968265042099,19.9411937080205));
#5450=CARTESIAN_POINT('Ctrl Pts',(6.51980121150529,-3.71512012776234,20.0173254587042));
#5451=CARTESIAN_POINT('Ctrl Pts',(6.39173197781128,-3.92374340698073,20.0969476480743));
#5452=CARTESIAN_POINT('Ctrl Pts',(6.24643834821673,-4.16042502504972,20.1872784524069));
#5453=CARTESIAN_POINT('Ctrl Pts',(6.08843156266247,-4.38833802903066,20.2821017096938));
#5454=CARTESIAN_POINT('Ctrl Pts',(5.91853733545478,-4.60661652504611,20.3790015676319));
#5455=CARTESIAN_POINT('Ctrl Pts',(5.73914601792361,-4.83709679287217,20.4813181293528));
#5456=CARTESIAN_POINT('Ctrl Pts',(5.5464996275473,-5.05683827770826,20.5859499447384));
#5457=CARTESIAN_POINT('Ctrl Pts',(5.34151401399943,-5.26481035159365,20.6900529536791));
#5458=CARTESIAN_POINT('Ctrl Pts',(5.15206615048807,-5.4570183040723,20.7862650355299));
#5459=CARTESIAN_POINT('Ctrl Pts',(4.95207643611402,-5.63917484269083,20.8820254389011));
#5460=CARTESIAN_POINT('Ctrl Pts',(4.74225084095691,-5.81042657310489,20.9750890530894));
#5461=CARTESIAN_POINT('Ctrl Pts',(4.72504179152039,-5.82447194965955,20.9827217555541));
#5462=CARTESIAN_POINT('Ctrl Pts',(4.70776658093554,-5.83844394397119,20.9903363177451));
#5463=CARTESIAN_POINT('Ctrl Pts',(4.69042560048463,-5.85234206846442,20.9979315010569));
#5464=CARTESIAN_POINT('Ctrl Pts',(4.53227676895431,-5.97909223436701,21.0671991742096));
#5465=CARTESIAN_POINT('Ctrl Pts',(4.36871099115427,-6.09965023465495,21.1348550392648));
#5466=CARTESIAN_POINT('Ctrl Pts',(4.20020516145961,-6.21355587418735,21.2001827671395));
#5467=CARTESIAN_POINT('Ctrl Pts',(4.03232824561985,-6.3270363840077,21.2652666725113));
#5468=CARTESIAN_POINT('Ctrl Pts',(3.85954822864127,-6.43391388412784,21.3280397868718));
#5469=CARTESIAN_POINT('Ctrl Pts',(3.6823763884026,-6.53376645849353,21.3877937718994));
#5470=CARTESIAN_POINT('Ctrl Pts',(3.50620389868854,-6.63305580722221,21.4472107102709));
#5471=CARTESIAN_POINT('Ctrl Pts',(3.32568916106491,-6.72539906465887,21.5036424824856));
#5472=CARTESIAN_POINT('Ctrl Pts',(3.14137181717059,-6.81041724905944,21.5563926690391));
#5473=CARTESIAN_POINT('Ctrl Pts',(2.95767572458469,-6.89514887519489,21.6089650583124));
#5474=CARTESIAN_POINT('Ctrl Pts',(2.77020278725585,-6.97260452982804,21.6578806380559));
#5475=CARTESIAN_POINT('Ctrl Pts',(2.57952150493091,-7.04244764308539,21.7024500070124));
#5476=CARTESIAN_POINT('Ctrl Pts',(2.38980714723273,-7.11193658929816,21.7467933694101));
#5477=CARTESIAN_POINT('Ctrl Pts',(2.196917093991,-7.17388983260061,21.7868344876134));
#5478=CARTESIAN_POINT('Ctrl Pts',(2.00144251249453,-7.2280168697354,21.8218943949161));
#5479=CARTESIAN_POINT('Ctrl Pts',(1.89911448599971,-7.25635156597884,21.8402477332167));
#5480=CARTESIAN_POINT('Ctrl Pts',(1.79607870623633,-7.2825422915802,21.8572360372855));
#5481=CARTESIAN_POINT('Ctrl Pts',(1.69242314334617,-7.30655212147743,21.872761906575));
#5482=CARTESIAN_POINT('Ctrl Pts',(1.53109479348353,-7.34392075013372,21.8969261945575));
#5483=CARTESIAN_POINT('Ctrl Pts',(1.3681702033035,-7.37602484342661,21.9175479596803));
#5484=CARTESIAN_POINT('Ctrl Pts',(1.20409713062058,-7.40271234751367,21.9346299924873));
#5485=CARTESIAN_POINT('Ctrl Pts',(1.04013459995097,-7.42938187125585,21.9517005165057));
#5486=CARTESIAN_POINT('Ctrl Pts',(0.875025527419233,-7.45064197717302,21.9652360762951));
#5487=CARTESIAN_POINT('Ctrl Pts',(0.709231910677198,-7.46639070079226,21.9752394567629));
#5488=CARTESIAN_POINT('Ctrl Pts',(0.543509118740266,-7.48213269676841,21.9852385639209));
#5489=CARTESIAN_POINT('Ctrl Pts',(0.377102774307521,-7.49236794293203,21.9917085089118));
#5490=CARTESIAN_POINT('Ctrl Pts',(0.210483412612377,-7.49704586707425,21.9946520730754));
#5491=CARTESIAN_POINT('Ctrl Pts',(0.043846333176655,-7.50172428865113,21.9975959502477));
#5492=CARTESIAN_POINT('Ctrl Pts',(-0.123003394892105,-7.50084417941287,
21.997012696586));
#5493=CARTESIAN_POINT('Ctrl Pts',(-0.289592115445145,-7.49440700834109,
21.9929050943176));
#5494=CARTESIAN_POINT('Ctrl Pts',(-0.456183318161168,-7.4879697413558,21.9887974308462));
#5495=CARTESIAN_POINT('Ctrl Pts',(-0.622513091568758,-7.47597527450695,
21.981165313742));
#5496=CARTESIAN_POINT('Ctrl Pts',(-0.788111005271544,-7.45847712628857,
21.9700115253567));
#5497=CARTESIAN_POINT('Ctrl Pts',(-0.953837293941331,-7.44096541313964,
21.9588490903214));
#5498=CARTESIAN_POINT('Ctrl Pts',(-1.11883017932857,-7.41794155647566,21.9441595217421));
#5499=CARTESIAN_POINT('Ctrl Pts',(-1.28262756847188,-7.38951057381989,21.9259456084462));
#5500=CARTESIAN_POINT('Ctrl Pts',(-1.42017866615189,-7.36563526730324,21.9106502256566));
#5501=CARTESIAN_POINT('Ctrl Pts',(-1.55688674308031,-7.33794777473905,21.8928694642867));
#5502=CARTESIAN_POINT('Ctrl Pts',(-1.69248640459601,-7.3065374679295,21.8726049758912));
#5503=CARTESIAN_POINT('Ctrl Pts',(-1.88273274116687,-7.2624688048201,21.844173896959));
#5504=CARTESIAN_POINT('Ctrl Pts',(-2.07088280936276,-7.21105234060234,21.8108538268066));
#5505=CARTESIAN_POINT('Ctrl Pts',(-2.25637490010937,-7.15253607541803,21.7732157763905));
#5506=CARTESIAN_POINT('Ctrl Pts',(-2.44228818762723,-7.09388693738798,21.7354922612775));
#5507=CARTESIAN_POINT('Ctrl Pts',(-2.62553116371187,-7.02810591273327,21.693431133967));
#5508=CARTESIAN_POINT('Ctrl Pts',(-2.80556734618175,-6.95548645790061,21.6476073040373));
#5509=CARTESIAN_POINT('Ctrl Pts',(-2.98633240777209,-6.8825730021419,21.6015979556612));
#5510=CARTESIAN_POINT('Ctrl Pts',(-3.16386441742821,-6.80276583871935,21.5517953762802));
#5511=CARTESIAN_POINT('Ctrl Pts',(-3.33765331847507,-6.716403079452,21.4987814863694));
#5512=CARTESIAN_POINT('Ctrl Pts',(-3.48618474969516,-6.64259178217798,21.4534723274095));
#5513=CARTESIAN_POINT('Ctrl Pts',(-3.63198249097864,-6.5639926901194,21.4058174549831));
#5514=CARTESIAN_POINT('Ctrl Pts',(-3.77474896103915,-6.48083870198402,21.3561801584053));
#5515=CARTESIAN_POINT('Ctrl Pts',(-4.01014670256992,-6.34373185190885,21.2743366589818));
#5516=CARTESIAN_POINT('Ctrl Pts',(-4.23726216824446,-6.19427134778842,21.1871036565295));
#5517=CARTESIAN_POINT('Ctrl Pts',(-4.45518879445125,-6.03334839088512,21.0965474453963));
#5518=CARTESIAN_POINT('Ctrl Pts',(-4.70496196761567,-5.84890907623891,20.9927578690687));
#5519=CARTESIAN_POINT('Ctrl Pts',(-4.94266540081088,-5.64941169864884,20.8846028468938));
#5520=CARTESIAN_POINT('Ctrl Pts',(-5.16700270581407,-5.43618276349407,20.775193369301));
#5521=CARTESIAN_POINT('Ctrl Pts',(-5.41937829936577,-5.19630389416685,20.6521095966433));
#5522=CARTESIAN_POINT('Ctrl Pts',(-5.65484050194211,-4.93904334303755,20.5274382025953));
#5523=CARTESIAN_POINT('Ctrl Pts',(-5.87159479072483,-4.66630202768028,20.405608498822));
#5524=CARTESIAN_POINT('Ctrl Pts',(-6.04218384490524,-4.45165029790822,20.3097265946877));
#5525=CARTESIAN_POINT('Ctrl Pts',(-6.20118676076994,-4.22740917015755,20.2156048161748));
#5526=CARTESIAN_POINT('Ctrl Pts',(-6.34773101513702,-3.99453513684228,20.1254023322322));
#5527=CARTESIAN_POINT('Ctrl Pts',(-6.49297957996139,-3.76372008871914,20.0359973849496));
#5528=CARTESIAN_POINT('Ctrl Pts',(-6.62598930102868,-3.52442256522106,19.9504427327492));
#5529=CARTESIAN_POINT('Ctrl Pts',(-6.74590126628717,-3.27762354542207,19.8708407777669));
#5530=CARTESIAN_POINT('Ctrl Pts',(-6.82733214648403,-3.11002507957565,19.8167839766326));
#5531=CARTESIAN_POINT('Ctrl Pts',(-6.90272398004706,-2.93895680522367,19.7654723313743));
#5532=CARTESIAN_POINT('Ctrl Pts',(-6.97175686004025,-2.76488811427908,19.7175734145484));
#5533=CARTESIAN_POINT('Ctrl Pts',(-7.04065596082013,-2.5911567520471,19.6697673213077));
#5534=CARTESIAN_POINT('Ctrl Pts',(-7.10322050225642,-2.41443685134032,19.6253607422239));
#5535=CARTESIAN_POINT('Ctrl Pts',(-7.15917310915023,-2.23522714577742,19.5850173762919));
#5536=CARTESIAN_POINT('Ctrl Pts',(-7.21512240740766,-2.0560280373928,19.5446763959776));
#5537=CARTESIAN_POINT('Ctrl Pts',(-7.26446033922906,-1.87433969536736,19.5083981482907));
#5538=CARTESIAN_POINT('Ctrl Pts',(-7.30695362166136,-1.69068884508356,19.4768462144938));
#5539=CARTESIAN_POINT('Ctrl Pts',(-7.34944690409365,-1.50703799479976,19.4452942806969));
#5540=CARTESIAN_POINT('Ctrl Pts',(-7.38509535231297,-1.32142493703578,19.4184686607899));
#5541=CARTESIAN_POINT('Ctrl Pts',(-7.41371272123842,-1.13440014410596,19.3970329360355));
#5542=CARTESIAN_POINT('Ctrl Pts',(-7.43818802515262,-0.974445234960639,
19.3786998083692));
#5543=CARTESIAN_POINT('Ctrl Pts',(-7.45752405553203,-0.813425201482107,
19.364309229696));
#5544=CARTESIAN_POINT('Ctrl Pts',(-7.47162453316991,-0.651787415752647,
19.3538503606095));
#5545=CARTESIAN_POINT('Ctrl Pts',(-7.48571915884413,-0.490216712747107,
19.3433958321506));
#5546=CARTESIAN_POINT('Ctrl Pts',(-7.49458250514591,-0.328029183151691,
19.3368697504885));
#5547=CARTESIAN_POINT('Ctrl Pts',(-7.49816978215991,-0.165680167503408,
19.3342612897069));
#5548=CARTESIAN_POINT('Ctrl Pts',(-7.49938932726501,-0.110487343927736,
19.3333745069004));
#5549=CARTESIAN_POINT('Ctrl Pts',(-7.4999995298899,-0.0552759010908673,
19.3329405052157));
#5550=CARTESIAN_POINT('Ctrl Pts',(-7.49999999972844,-6.38227930839602E-5,
19.332958859286));
#5551=CARTESIAN_POINT('Ctrl Pts',(-7.49999999972845,-6.38221443329073E-5,
19.3329588592862));
#5552=CARTESIAN_POINT('Ctrl Pts',(-7.50000137686945,0.161769623405833,19.3330126573518));
#5553=CARTESIAN_POINT('Ctrl Pts',(-7.4947604010034,0.323599227211819,19.3369528643072));
#5554=CARTESIAN_POINT('Ctrl Pts',(-7.48430383616557,0.48497019285453,19.3447687682629));
#5555=CARTESIAN_POINT('Ctrl Pts',(-7.47384231895815,0.646417585954605,19.3525883739357));
#5556=CARTESIAN_POINT('Ctrl Pts',(-7.45816032347053,0.807405489160749,19.3642873486424));
#5557=CARTESIAN_POINT('Ctrl Pts',(-7.43733642357596,0.967484843576559,19.3798549652665));
#5558=CARTESIAN_POINT('Ctrl Pts',(-7.43007828607042,1.02328025039424,19.385281033518));
#5559=CARTESIAN_POINT('Ctrl Pts',(-7.42219593523814,1.07896536718678,19.3911770876185));
#5560=CARTESIAN_POINT('Ctrl Pts',(-7.4136941505238,1.13452150375796,19.3975426733416));
#5561=CARTESIAN_POINT('Ctrl Pts',(-7.38485140438262,1.32299858210651,19.4191382534722));
#5562=CARTESIAN_POINT('Ctrl Pts',(-7.34886996628597,1.5100294373421,19.4461378648968));
#5563=CARTESIAN_POINT('Ctrl Pts',(-7.30594116139313,1.69505862620195,19.4778961232255));
#5564=CARTESIAN_POINT('Ctrl Pts',(-7.26293850090524,1.88040614306737,19.5097090191122));
#5565=CARTESIAN_POINT('Ctrl Pts',(-7.21296472182939,2.06374480770197,19.546296949735));
#5566=CARTESIAN_POINT('Ctrl Pts',(-7.15625861648385,2.2445406242705,19.5870111939725));
#5567=CARTESIAN_POINT('Ctrl Pts',(-7.09936154725929,2.42594529010196,19.6278625477851));
#5568=CARTESIAN_POINT('Ctrl Pts',(-7.03568692374006,2.60478967078624,19.6728680536135));
#5569=CARTESIAN_POINT('Ctrl Pts',(-6.96551997668802,2.78056315417582,19.7213724143269));
#5570=CARTESIAN_POINT('Ctrl Pts',(-6.89820683644311,2.94918763672547,19.7679040217627));
#5571=CARTESIAN_POINT('Ctrl Pts',(-6.82491919803976,3.11498593049364,19.8176556633038));
#5572=CARTESIAN_POINT('Ctrl Pts',(-6.7459440810335,3.27753542399913,19.8700487900425));
#5573=CARTESIAN_POINT('Ctrl Pts',(-6.63072214042775,3.51468946436221,19.9464885341807));
#5574=CARTESIAN_POINT('Ctrl Pts',(-6.50338764282049,3.74495378726884,20.0285508887797));
#5575=CARTESIAN_POINT('Ctrl Pts',(-6.36470549534165,3.96743291784093,20.1143153130233));
#5576=CARTESIAN_POINT('Ctrl Pts',(-6.2136393301195,4.20977895666768,20.207738316045));
#5577=CARTESIAN_POINT('Ctrl Pts',(-6.0491079526643,4.44288805980257,20.3055540831348));
#5578=CARTESIAN_POINT('Ctrl Pts',(-5.87210066028485,4.66566542258253,20.4052802616237));
#5579=CARTESIAN_POINT('Ctrl Pts',(-5.67438099506923,4.91451090795411,20.5166758225579));
#5580=CARTESIAN_POINT('Ctrl Pts',(-5.46109323358007,5.15046648299211,20.6304550435319));
#5581=CARTESIAN_POINT('Ctrl Pts',(-5.23363288347398,5.37206541667354,20.7431582152801));
#5582=CARTESIAN_POINT('Ctrl Pts',(-5.01495184833834,5.58511126919161,20.8515113689153));
#5583=CARTESIAN_POINT('Ctrl Pts',(-4.78316943962577,5.78488927769216,20.9588699351008));
#5584=CARTESIAN_POINT('Ctrl Pts',(-4.53956528780731,5.97012118786,21.0621595457893));
#5585=CARTESIAN_POINT('Ctrl Pts',(-4.3266267571509,6.13203554969409,21.1524467505347));
#5586=CARTESIAN_POINT('Ctrl Pts',(-4.10465503258614,6.28283627218151,21.2396249456005));
#5587=CARTESIAN_POINT('Ctrl Pts',(-3.87454829813565,6.42167232778302,21.3216407735323));
#5588=CARTESIAN_POINT('Ctrl Pts',(-3.84141025626157,6.44166633202258,21.3334520051629));
#5589=CARTESIAN_POINT('Ctrl Pts',(-3.8081035883213,6.46141219329767,21.3451561726828));
#5590=CARTESIAN_POINT('Ctrl Pts',(-3.77463107174321,6.48090736488578,21.3567471433162));
#5591=CARTESIAN_POINT('Ctrl Pts',(-3.59538368742212,6.58530520739359,21.4188175037246));
#5592=CARTESIAN_POINT('Ctrl Pts',(-3.41138061249562,6.68250937266347,21.4776417528438));
#5593=CARTESIAN_POINT('Ctrl Pts',(-3.22316644017786,6.77208964049585,21.5326304570881));
#5594=CARTESIAN_POINT('Ctrl Pts',(-3.03610753231628,6.86112006185212,21.5872816389518));
#5595=CARTESIAN_POINT('Ctrl Pts',(-2.8448891541714,6.9426196918104,21.6381442168227));
#5596=CARTESIAN_POINT('Ctrl Pts',(-2.65008522422012,7.0161989926434,21.6846395445151));
#5597=CARTESIAN_POINT('Ctrl Pts',(-2.45716260701487,7.08906770372322,21.7306858450619));
#5598=CARTESIAN_POINT('Ctrl Pts',(-2.26072348245475,7.15416815105665,21.7724488412702));
#5599=CARTESIAN_POINT('Ctrl Pts',(-2.06136233189299,7.2111570040218,21.8093664903413));
#5600=CARTESIAN_POINT('Ctrl Pts',(-1.93952212373797,7.24598592474294,21.8319288302693));
#5601=CARTESIAN_POINT('Ctrl Pts',(-1.81659123049385,7.2777857918624,21.8526813930556));
#5602=CARTESIAN_POINT('Ctrl Pts',(-1.69271195884026,7.30648521687406,21.871495880758));
#5603=CARTESIAN_POINT('Ctrl Pts',(-1.54076476717671,7.34168720809236,21.8945732570681));
#5604=CARTESIAN_POINT('Ctrl Pts',(-1.3873755369066,7.37222456154265,21.9147348270972));
#5605=CARTESIAN_POINT('Ctrl Pts',(-1.23296187718936,7.39795951660981,21.9318611863869));
#5606=CARTESIAN_POINT('Ctrl Pts',(-1.07863059043489,7.4236807431992,21.9489784095097));
#5607=CARTESIAN_POINT('Ctrl Pts',(-0.923276373536958,7.44460457864745,21.9630636593349));
#5608=CARTESIAN_POINT('Ctrl Pts',(-0.767329781169641,7.46064373944569,21.9739977223933));
#5609=CARTESIAN_POINT('Ctrl Pts',(-0.611426078689014,7.4766784890043,21.9849287782638));
#5610=CARTESIAN_POINT('Ctrl Pts',(-0.454930745505132,7.4878311887663,21.9927103804668));
#5611=CARTESIAN_POINT('Ctrl Pts',(-0.298281394079239,7.49406619999758,21.9972234138677));
#5612=CARTESIAN_POINT('Ctrl Pts',(-0.141560740138866,7.500304049236,22.0017385014785));
#5613=CARTESIAN_POINT('Ctrl Pts',(0.0153136481942017,7.50161972110047,22.0029820440832));
#5614=CARTESIAN_POINT('Ctrl Pts',(0.171902471705738,7.49802971054539,22.0008347638195));
#5615=CARTESIAN_POINT('Ctrl Pts',(0.305568621085933,7.49496523329619,21.9990018189256));
#5616=CARTESIAN_POINT('Ctrl Pts',(0.439026530392158,7.48832709367931,21.9946981373927));
#5617=CARTESIAN_POINT('Ctrl Pts',(0.572005831492304,7.47815547636841,21.9878495298179));
#5618=CARTESIAN_POINT('Ctrl Pts',(0.768094469245658,7.4631566113891,21.9777507090335));
#5619=CARTESIAN_POINT('Ctrl Pts',(0.963317829131666,7.44046192620981,21.9621182351183));
#5620=CARTESIAN_POINT('Ctrl Pts',(1.15706933924185,7.41020853580966,21.9414600255889));
#5621=CARTESIAN_POINT('Ctrl Pts',(1.35121737676857,7.37989322951153,21.9207595374395));
#5622=CARTESIAN_POINT('Ctrl Pts',(1.54388725002921,7.34198837015578,21.8950127215142));
#5623=CARTESIAN_POINT('Ctrl Pts',(1.73448713276613,7.29668105279851,21.8647306201931));
#5624=CARTESIAN_POINT('Ctrl Pts',(1.92549417720536,7.25127694941914,21.8343838298924));
#5625=CARTESIAN_POINT('Ctrl Pts',(2.11442210634573,7.19843887574435,21.79948235684));
#5626=CARTESIAN_POINT('Ctrl Pts',(2.30069800903712,7.13840238927539,21.7605405255016));
#5627=CARTESIAN_POINT('Ctrl Pts',(2.48738865405972,7.0782322318807,21.7215119903777));
#5628=CARTESIAN_POINT('Ctrl Pts',(2.67141519319667,7.01083174340814,21.6784250852651));
#5629=CARTESIAN_POINT('Ctrl Pts',(2.85222764907197,6.93648307414279,21.6317975777061));
#5630=CARTESIAN_POINT('Ctrl Pts',(3.03371105458721,6.86185851562726,21.5849970471701));
#5631=CARTESIAN_POINT('Ctrl Pts',(3.21195623090598,6.78023430023224,21.5346295888609));
#5632=CARTESIAN_POINT('Ctrl Pts',(3.38643781016122,6.69193835580622,21.4812187556522));
#5633=CARTESIAN_POINT('Ctrl Pts',(3.56127443599491,6.60346274099269,21.4276992385717));
#5634=CARTESIAN_POINT('Ctrl Pts',(3.73233191190736,6.50828843639492,21.3711239482717));
#5635=CARTESIAN_POINT('Ctrl Pts',(3.89911599643454,6.40678503200695,21.3120196402132));
#5636=CARTESIAN_POINT('Ctrl Pts',(4.0664769606818,6.30493054342724,21.2527108997186));
#5637=CARTESIAN_POINT('Ctrl Pts',(4.229534712043,6.19670332730237,21.190855616266));
#5638=CARTESIAN_POINT('Ctrl Pts',(4.38782764842825,6.08251333970495,21.1269860301346));
#5639=CARTESIAN_POINT('Ctrl Pts',(4.49080837173162,6.00822469622331,21.0854343581075));
#5640=CARTESIAN_POINT('Ctrl Pts',(4.59177320403997,5.93141309365973,21.0430301484942));
#5641=CARTESIAN_POINT('Ctrl Pts',(4.69060418288513,5.85219893710907,20.9999199530233));
#5642=CARTESIAN_POINT('Ctrl Pts',(4.90988924268625,5.67643946108971,20.9042675381394));
#5643=CARTESIAN_POINT('Ctrl Pts',(5.11865959298013,5.48887002871858,20.8051395384096));
#5644=CARTESIAN_POINT('Ctrl Pts',(5.31613179428595,5.29043880465336,20.7051913113127));
#5645=CARTESIAN_POINT('Ctrl Pts',(5.51624645380641,5.08935228928837,20.603905635137));
#5646=CARTESIAN_POINT('Ctrl Pts',(5.70476104395003,4.87710926925346,20.5017776331107));
#5647=CARTESIAN_POINT('Ctrl Pts',(5.88083921476348,4.65464608000438,20.4015706928499));
#5648=CARTESIAN_POINT('Ctrl Pts',(6.04863046411871,4.44265287103811,20.3060798797483));
#5649=CARTESIAN_POINT('Ctrl Pts',(6.20512960953633,4.22137645327274,20.2123335583494));
#5650=CARTESIAN_POINT('Ctrl Pts',(6.34956762900155,3.99161507722572,20.1227230237679));
#5651=CARTESIAN_POINT('Ctrl Pts',(6.4782693500351,3.78688584711183,20.0428754180885));
#5652=CARTESIAN_POINT('Ctrl Pts',(6.59739471133209,3.57541842759605,19.966311514912));
#5653=CARTESIAN_POINT('Ctrl Pts',(6.70635739485687,3.35779250288766,19.8947230855874));
#5654=CARTESIAN_POINT('Ctrl Pts',(6.71968021052779,3.33118348421894,19.8859700022637));
#5655=CARTESIAN_POINT('Ctrl Pts',(6.73285104073735,3.30448243080959,19.8772913014631));
#5656=CARTESIAN_POINT('Ctrl Pts',(6.74586876681577,3.27769043396406,19.8686900755905));
#5657=CARTESIAN_POINT('Ctrl Pts',(6.82430646662419,3.11625650969972,19.8168637912674));
#5658=CARTESIAN_POINT('Ctrl Pts',(6.89715640692234,2.9515711207856,19.7678503184023));
#5659=CARTESIAN_POINT('Ctrl Pts',(6.96411695834188,2.78407524871995,19.7220840532085));
#5660=CARTESIAN_POINT('Ctrl Pts',(7.03097289981926,2.61684104913335,19.6763892869234));
#5661=CARTESIAN_POINT('Ctrl Pts',(7.09195760838124,2.44680543583005,19.633931590255));
#5662=CARTESIAN_POINT('Ctrl Pts',(7.14681265559779,2.27443814287996,19.5951433266732));
#5663=CARTESIAN_POINT('Ctrl Pts',(7.20159314251032,2.10230513571426,19.5564077850354));
#5664=CARTESIAN_POINT('Ctrl Pts',(7.25026042307138,1.92784710265306,19.5213317080993));
#5665=CARTESIAN_POINT('Ctrl Pts',(7.29260203951382,1.75155801881608,19.4903456986937));
#5666=CARTESIAN_POINT('Ctrl Pts',(7.33488204075116,1.57552546954176,19.4594047798984));
#5667=CARTESIAN_POINT('Ctrl Pts',(7.37085461729061,1.39766753541784,19.4325420336229));
#5668=CARTESIAN_POINT('Ctrl Pts',(7.40035570833137,1.21849718512899,19.4101861855999));
#5669=CARTESIAN_POINT('Ctrl Pts',(7.42983195743503,1.03947770853382,19.3878491627305));
#5670=CARTESIAN_POINT('Ctrl Pts',(7.45284749385224,0.859148380629525,19.3700114510759));
#5671=CARTESIAN_POINT('Ctrl Pts',(7.46928819351229,0.678036785327972,19.3571006942315));
#5672=CARTESIAN_POINT('Ctrl Pts',(7.48571612175541,0.497065880613931,19.3441999666841));
#5673=CARTESIAN_POINT('Ctrl Pts',(7.49557934457186,0.315314290784328,19.3362185422342));
#5674=CARTESIAN_POINT('Ctrl Pts',(7.49881497880803,0.133318841895481,19.3335830686486));
#5675=CARTESIAN_POINT('Ctrl Pts',(7.49960484421833,0.0888911039569122,19.3329397111881));
#5676=CARTESIAN_POINT('Ctrl Pts',(7.5,0.0444488682210776,19.3326149291812));
#5677=CARTESIAN_POINT('Ctrl Pts',(7.5,1.83697019872103E-15,19.3326149291812));
#5678=CARTESIAN_POINT('Ctrl Pts',(9.06818181818182,-2.77555756156289E-16,
16.6963492570201));
#5679=CARTESIAN_POINT('Ctrl Pts',(9.06818181818182,-1.59578114831733,16.6963492570201));
#5680=CARTESIAN_POINT('Ctrl Pts',(8.41792693003091,-4.7680728734062,17.0694389926071));
#5681=CARTESIAN_POINT('Ctrl Pts',(5.86812439794336,-8.45147311504401,18.176238977512));
#5682=CARTESIAN_POINT('Ctrl Pts',(2.13637643354675,-10.5855566851176,19.0330683300942));
#5683=CARTESIAN_POINT('Ctrl Pts',(-1.66033921810787,-10.5859872665705,19.0322636243943));
#5684=CARTESIAN_POINT('Ctrl Pts',(-5.48966678697824,-8.80610845315595,18.3204282727391));
#5685=CARTESIAN_POINT('Ctrl Pts',(-7.9972027779537,-5.6823888865083,17.2720041386699));
#5686=CARTESIAN_POINT('Ctrl Pts',(-9.10276599747076,-1.62090974430359,16.6774277042663));
#5687=CARTESIAN_POINT('Ctrl Pts',(-9.10168338064412,1.6211254766953,16.678827094141));
#5688=CARTESIAN_POINT('Ctrl Pts',(-7.99795456455011,5.6815718382537,17.2694619372668));
#5689=CARTESIAN_POINT('Ctrl Pts',(-5.48802720874369,8.80873683615948,18.3244182502819));
#5690=CARTESIAN_POINT('Ctrl Pts',(-2.08802932955049,10.3840276033752,18.9482929035547));
#5691=CARTESIAN_POINT('Ctrl Pts',(1.64285450861998,10.7207692947679,19.0979776863544));
#5692=CARTESIAN_POINT('Ctrl Pts',(5.59169260247156,8.86861695682125,18.3071970067273));
#5693=CARTESIAN_POINT('Ctrl Pts',(8.41406720829093,4.76388507099759,17.0652606363946));
#5694=CARTESIAN_POINT('Ctrl Pts',(9.06818181818182,1.59578114831733,16.6963492570201));
#5695=CARTESIAN_POINT('Ctrl Pts',(9.06818181818182,-2.77555756156289E-16,
16.6963492570201));
#5696=CARTESIAN_POINT('Ctrl Pts',(8.52925489606833,-2.04324230714416E-16,
16.9890532033264));
#5697=CARTESIAN_POINT('Ctrl Pts',(8.52925489606833,-1.48962154953277,16.9890532033264));
#5698=CARTESIAN_POINT('Ctrl Pts',(7.87687500329371,-4.44985072056414,17.3363463617318));
#5699=CARTESIAN_POINT('Ctrl Pts',(5.37101016546914,-7.81747651588321,18.3271776375016));
#5700=CARTESIAN_POINT('Ctrl Pts',(1.90652317397209,-9.67880593256366,19.027936254452));
#5701=CARTESIAN_POINT('Ctrl Pts',(-1.48242488666645,-9.67656253638176,19.0242925274118));
#5702=CARTESIAN_POINT('Ctrl Pts',(-5.00803293593842,-8.13057125719761,18.4491055978167));
#5703=CARTESIAN_POINT('Ctrl Pts',(-7.45861508030558,-5.2962344172881,17.5218568938428));
#5704=CARTESIAN_POINT('Ctrl Pts',(-8.56396284436833,-1.5139035461346,16.9719681314427));
#5705=CARTESIAN_POINT('Ctrl Pts',(-8.56304269786486,1.51420311672056,16.9729380768753));
#5706=CARTESIAN_POINT('Ctrl Pts',(-7.45892636451772,5.29539679129704,17.5194393239992));
#5707=CARTESIAN_POINT('Ctrl Pts',(-5.00753889620558,8.13267896507007,18.4521891181082));
#5708=CARTESIAN_POINT('Ctrl Pts',(-1.87388181025726,9.50233127388934,18.9572985482202));
#5709=CARTESIAN_POINT('Ctrl Pts',(1.46541943459002,9.79166364559922,19.0778999502934));
#5710=CARTESIAN_POINT('Ctrl Pts',(5.0943002984368,8.19665431249147,18.4428143198929));
#5711=CARTESIAN_POINT('Ctrl Pts',(7.87606641456947,4.44699289538305,17.3333349814256));
#5712=CARTESIAN_POINT('Ctrl Pts',(8.52925489606833,1.48962154953272,16.9890532033264));
#5713=CARTESIAN_POINT('Ctrl Pts',(8.52925489606833,-2.41380287841585E-16,
16.9890532033264));
#5714=CARTESIAN_POINT('Ctrl Pts',(7.75033632345811,-4.50174017686739E-17,
17.7987073905814));
#5715=CARTESIAN_POINT('Ctrl Pts',(7.75033632345811,-1.30455312354164,17.7987073905814));
#5716=CARTESIAN_POINT('Ctrl Pts',(7.10826290029318,-3.89360315842007,18.1503268520871));
#5717=CARTESIAN_POINT('Ctrl Pts',(4.70053765930092,-6.71224153203073,19.133184606454));
#5718=CARTESIAN_POINT('Ctrl Pts',(1.60333612140186,-8.1097961186631,19.7809692603298));
#5719=CARTESIAN_POINT('Ctrl Pts',(-1.24739767962264,-8.10458971579584,19.7768036158037));
#5720=CARTESIAN_POINT('Ctrl Pts',(-4.36061605167524,-6.95356866926854,19.2482436597623));
#5721=CARTESIAN_POINT('Ctrl Pts',(-6.70160515983065,-4.62154273010426,18.3373097614389));
#5722=CARTESIAN_POINT('Ctrl Pts',(-7.78395626574493,-1.32716243511598,17.7808035499084));
#5723=CARTESIAN_POINT('Ctrl Pts',(-7.78335904380905,1.32737409349607,17.7818079474956));
#5724=CARTESIAN_POINT('Ctrl Pts',(-6.70129128714702,4.62079718556549,18.3348534089681));
#5725=CARTESIAN_POINT('Ctrl Pts',(-4.36163002862514,6.95584707246026,19.2523271250457));
#5726=CARTESIAN_POINT('Ctrl Pts',(-1.59115196857109,7.97628900960331,19.7149140395441));
#5727=CARTESIAN_POINT('Ctrl Pts',(1.2323404820187,8.1853538169283,19.8249773268813));
#5728=CARTESIAN_POINT('Ctrl Pts',(4.42748256065924,7.02563177285682,19.2467581349916));
#5729=CARTESIAN_POINT('Ctrl Pts',(7.11158331347841,3.89285136784028,18.1476536477004));
#5730=CARTESIAN_POINT('Ctrl Pts',(7.75033632345811,1.30455312354152,17.7987073905814));
#5731=CARTESIAN_POINT('Ctrl Pts',(7.75033632345811,-1.62495706346568E-16,
17.7987073905814));
#5732=CARTESIAN_POINT('Ctrl Pts',(7.49997898926977,1.18727990181773E-16,
18.8727417166749));
#5733=CARTESIAN_POINT('Ctrl Pts',(7.49997898926977,-1.17773001028884,18.8727417166749));
#5734=CARTESIAN_POINT('Ctrl Pts',(6.92434994470585,-3.5173122090396,19.2806044731049));
#5735=CARTESIAN_POINT('Ctrl Pts',(4.71974380892434,-6.14234789882435,20.4728855461179));
#5736=CARTESIAN_POINT('Ctrl Pts',(1.6753432303372,-7.55890683324212,21.3625000258593));
#5737=CARTESIAN_POINT('Ctrl Pts',(-1.30266100196853,-7.55659632853009,21.3607622545602));
#5738=CARTESIAN_POINT('Ctrl Pts',(-4.40054398399628,-6.38168901511819,20.6242901562785));
#5739=CARTESIAN_POINT('Ctrl Pts',(-6.55612322809675,-4.18225627169105,19.5009453626012));
#5740=CARTESIAN_POINT('Ctrl Pts',(-7.53043693696764,-1.19744723403944,18.851946280041));
#5741=CARTESIAN_POINT('Ctrl Pts',(-7.52965797516887,1.19768815648017,18.8534063249902));
#5742=CARTESIAN_POINT('Ctrl Pts',(-6.55645674912434,4.18156062850628,19.4981462935819));
#5743=CARTESIAN_POINT('Ctrl Pts',(-4.40001770889782,6.38344201396891,20.628879238981));
#5744=CARTESIAN_POINT('Ctrl Pts',(-1.64701789222801,7.42449614751224,21.2739304159005));
#5745=CARTESIAN_POINT('Ctrl Pts',(1.28815795162506,7.64293786766958,21.4284314886368));
#5746=CARTESIAN_POINT('Ctrl Pts',(4.47613818554217,6.43700979105439,20.6131496315766));
#5747=CARTESIAN_POINT('Ctrl Pts',(6.92370291988582,3.51549848232719,19.2763960689845));
#5748=CARTESIAN_POINT('Ctrl Pts',(7.49997898926977,1.17773001028865,18.8727417166749));
#5749=CARTESIAN_POINT('Ctrl Pts',(7.49997898926977,-8.11489720641551E-17,
18.8727417166749));
#5750=CARTESIAN_POINT('Ctrl Pts',(7.50000000308588,1.82342057246943E-16,
19.3327500340666));
#5751=CARTESIAN_POINT('Ctrl Pts',(7.50000000308588,-1.13983254637561,19.3327500340666));
#5752=CARTESIAN_POINT('Ctrl Pts',(6.96220632038699,-3.40573356596564,19.7647557660862));
#5753=CARTESIAN_POINT('Ctrl Pts',(4.85337521228726,-6.03673548829487,21.0463398717424));
#5754=CARTESIAN_POINT('Ctrl Pts',(1.76695478202178,-7.56111255891257,22.0384881837842));
#5755=CARTESIAN_POINT('Ctrl Pts',(-1.37323361305111,-7.56142088620697,22.037556656091));
#5756=CARTESIAN_POINT('Ctrl Pts',(-4.54036697665852,-6.29005054782313,21.2133004666028));
#5757=CARTESIAN_POINT('Ctrl Pts',(-6.61424492839959,-4.05881294736392,19.999309056778));
#5758=CARTESIAN_POINT('Ctrl Pts',(-7.52860291482921,-1.15778102404128,19.3108405405169));
#5759=CARTESIAN_POINT('Ctrl Pts',(-7.52770748324762,1.15793509310074,19.3124609337831));
#5760=CARTESIAN_POINT('Ctrl Pts',(-6.61486679147359,4.05822937438032,19.9963654126915));
#5761=CARTESIAN_POINT('Ctrl Pts',(-4.53901069073959,6.29192800079645,21.2179204496805));
#5762=CARTESIAN_POINT('Ctrl Pts',(-1.72696502969537,7.41716041273811,21.9403243457452));
#5763=CARTESIAN_POINT('Ctrl Pts',(1.35877258747706,7.6576966809742,22.1136490964728));
#5764=CARTESIAN_POINT('Ctrl Pts',(4.62475181174631,6.33469634386154,21.1979788253294));
#5765=CARTESIAN_POINT('Ctrl Pts',(6.95901332159314,3.40274193259946,19.7599174844227));
#5766=CARTESIAN_POINT('Ctrl Pts',(7.50000000308588,1.13983254637542,19.3327500340666));
#5767=CARTESIAN_POINT('Ctrl Pts',(7.50000000308588,-4.94995460683127E-17,
19.3327500340666));
#5768=CARTESIAN_POINT('',(9.06818181818182,-2.77555756156289E-16,16.6963492570201));
#5769=CARTESIAN_POINT('Ctrl Pts',(9.06818181818182,-2.77555756156289E-16,
16.6963492570201));
#5770=CARTESIAN_POINT('Ctrl Pts',(8.52925489606833,-2.04324230714416E-16,
16.9890532033264));
#5771=CARTESIAN_POINT('Ctrl Pts',(7.75036900658895,-4.50240862234006E-17,
17.7986734177958));
#5772=CARTESIAN_POINT('Ctrl Pts',(7.49999999999984,1.1871424879926E-16,
18.8726515849863));
#5773=CARTESIAN_POINT('Ctrl Pts',(7.5,1.82323373546833E-16,19.3326149291822));
#5774=CARTESIAN_POINT('Ctrl Pts',(9.06818181818182,-2.77555756156289E-16,
16.6963492570201));
#5775=CARTESIAN_POINT('Ctrl Pts',(9.06818181818182,1.59578114831733,16.6963492570201));
#5776=CARTESIAN_POINT('Ctrl Pts',(8.41406720829093,4.76388507099759,17.0652606363946));
#5777=CARTESIAN_POINT('Ctrl Pts',(5.59169260247156,8.86861695682125,18.3071970067273));
#5778=CARTESIAN_POINT('Ctrl Pts',(1.64285450861998,10.7207692947679,19.0979776863544));
#5779=CARTESIAN_POINT('Ctrl Pts',(-2.08802932955049,10.3840276033752,18.9482929035547));
#5780=CARTESIAN_POINT('Ctrl Pts',(-5.48802720874369,8.80873683615948,18.3244182502819));
#5781=CARTESIAN_POINT('Ctrl Pts',(-7.99795456455011,5.6815718382537,17.2694619372668));
#5782=CARTESIAN_POINT('Ctrl Pts',(-9.10168338064412,1.6211254766953,16.678827094141));
#5783=CARTESIAN_POINT('Ctrl Pts',(-9.10276599747076,-1.62090974430359,16.6774277042663));
#5784=CARTESIAN_POINT('Ctrl Pts',(-7.9972027779537,-5.6823888865083,17.2720041386699));
#5785=CARTESIAN_POINT('Ctrl Pts',(-5.48966678697824,-8.80610845315595,18.3204282727391));
#5786=CARTESIAN_POINT('Ctrl Pts',(-1.66033921810787,-10.5859872665705,19.0322636243943));
#5787=CARTESIAN_POINT('Ctrl Pts',(2.13637643354675,-10.5855566851176,19.0330683300942));
#5788=CARTESIAN_POINT('Ctrl Pts',(5.86812439794336,-8.45147311504401,18.176238977512));
#5789=CARTESIAN_POINT('Ctrl Pts',(8.41792693003091,-4.7680728734062,17.0694389926071));
#5790=CARTESIAN_POINT('Ctrl Pts',(9.06818181818182,-1.59578114831733,16.6963492570201));
#5791=CARTESIAN_POINT('Ctrl Pts',(9.06818181818182,-2.77555756156289E-16,
16.6963492570201));
#5792=CARTESIAN_POINT('Origin',(0.,0.,0.));
#5793=CARTESIAN_POINT('',(-19.,20.,2.32682891837997E-15));
#5794=CARTESIAN_POINT('Origin',(0.,20.,0.));
#5795=CARTESIAN_POINT('',(-19.,-20.,2.32682891837997E-15));
#5796=CARTESIAN_POINT('',(-19.,0.,2.32682891837997E-15));
#5797=CARTESIAN_POINT('Origin',(0.,-20.,0.));
#5798=CARTESIAN_POINT('Origin',(0.,0.,0.));
#5799=CARTESIAN_POINT('',(6.,6.93889390390723E-16,10.3923048454133));
#5800=CARTESIAN_POINT('',(-6.,-7.34788079488412E-16,10.3923048454133));
#5801=CARTESIAN_POINT('Ctrl Pts',(6.,5.55111512312578E-16,10.3923048454133));
#5802=CARTESIAN_POINT('Ctrl Pts',(6.,0.769830401762947,10.3923048454133));
#5803=CARTESIAN_POINT('Ctrl Pts',(5.84331350686056,1.57883160757971,10.4869526157176));
#5804=CARTESIAN_POINT('Ctrl Pts',(5.22737225841736,3.05149415704693,10.8071760747641));
#5805=CARTESIAN_POINT('Ctrl Pts',(4.76853496878621,3.71674640545236,11.026202805293));
#5806=CARTESIAN_POINT('Ctrl Pts',(3.71818001883758,4.76710135540099,11.423199660423));
#5807=CARTESIAN_POINT('Ctrl Pts',(3.05244454868625,5.22699047954748,11.6295890462369));
#5808=CARTESIAN_POINT('Ctrl Pts',(1.57767045293313,5.84378343521477,11.9195518101039));
#5809=CARTESIAN_POINT('Ctrl Pts',(0.767731806652134,6.,12.));
#5810=CARTESIAN_POINT('Ctrl Pts',(-0.767731806652134,6.,12.));
#5811=CARTESIAN_POINT('Ctrl Pts',(-1.57767045293313,5.84378343521477,11.9195518101039));
#5812=CARTESIAN_POINT('Ctrl Pts',(-3.05244454868625,5.22699047954748,11.6295890462369));
#5813=CARTESIAN_POINT('Ctrl Pts',(-3.71818001883758,4.76710135540099,11.423199660423));
#5814=CARTESIAN_POINT('Ctrl Pts',(-4.76853496878621,3.71674640545236,11.026202805293));
#5815=CARTESIAN_POINT('Ctrl Pts',(-5.22737225841736,3.05149415704693,10.8071760747641));
#5816=CARTESIAN_POINT('Ctrl Pts',(-5.84331350686056,1.57883160757971,10.4869526157176));
#5817=CARTESIAN_POINT('Ctrl Pts',(-6.,0.769830401762947,10.3923048454133));
#5818=CARTESIAN_POINT('Ctrl Pts',(-6.,5.55111512312578E-16,10.3923048454133));
#5819=CARTESIAN_POINT('Ctrl Pts',(-6.,-2.77555756156289E-16,10.3923048454133));
#5820=CARTESIAN_POINT('Ctrl Pts',(-6.,-0.769830401762946,10.3923048454133));
#5821=CARTESIAN_POINT('Ctrl Pts',(-5.84331350686056,-1.57883160757971,10.4869526157176));
#5822=CARTESIAN_POINT('Ctrl Pts',(-5.22737225841736,-3.05149415704693,10.8071760747641));
#5823=CARTESIAN_POINT('Ctrl Pts',(-4.76853496878621,-3.71674640545236,11.026202805293));
#5824=CARTESIAN_POINT('Ctrl Pts',(-3.71818001883758,-4.76710135540099,11.423199660423));
#5825=CARTESIAN_POINT('Ctrl Pts',(-3.05244454868625,-5.22699047954748,11.6295890462369));
#5826=CARTESIAN_POINT('Ctrl Pts',(-1.57767045293313,-5.84378343521477,11.9195518101039));
#5827=CARTESIAN_POINT('Ctrl Pts',(-0.767731806652135,-6.,12.));
#5828=CARTESIAN_POINT('Ctrl Pts',(0.767731806652132,-6.,12.));
#5829=CARTESIAN_POINT('Ctrl Pts',(1.57767045293313,-5.84378343521477,11.9195518101039));
#5830=CARTESIAN_POINT('Ctrl Pts',(3.05244454868625,-5.22699047954749,11.6295890462369));
#5831=CARTESIAN_POINT('Ctrl Pts',(3.71818001883758,-4.767101355401,11.423199660423));
#5832=CARTESIAN_POINT('Ctrl Pts',(4.76853496878621,-3.71674640545237,11.026202805293));
#5833=CARTESIAN_POINT('Ctrl Pts',(5.22737225841736,-3.05149415704693,10.8071760747641));
#5834=CARTESIAN_POINT('Ctrl Pts',(5.84331350686056,-1.57883160757971,10.4869526157176));
#5835=CARTESIAN_POINT('Ctrl Pts',(6.,-0.769830401762948,10.3923048454133));
#5836=CARTESIAN_POINT('Ctrl Pts',(6.,-8.32667268468867E-16,10.3923048454133));
#5837=CARTESIAN_POINT('',(-6.,-7.34788079488412E-16,0.));
#5838=CARTESIAN_POINT('Origin',(0.,20.,0.));
#5839=CARTESIAN_POINT('',(-15.,20.,-1.83697019872103E-15));
#5840=CARTESIAN_POINT('Origin',(0.,20.,0.));
#5841=CARTESIAN_POINT('',(-15.,26.,-1.83697019872103E-15));
#5842=CARTESIAN_POINT('',(-15.,20.,-1.83697019872103E-15));
#5843=CARTESIAN_POINT('Origin',(0.,26.,0.));
#5844=CARTESIAN_POINT('Origin',(0.,26.,0.));
#5845=CARTESIAN_POINT('',(-12.,26.,-1.46957615897682E-15));
#5846=CARTESIAN_POINT('Origin',(0.,26.,0.));
#5847=CARTESIAN_POINT('Origin',(0.,-20.,0.));
#5848=CARTESIAN_POINT('',(-15.,-26.,-1.83697019872103E-15));
#5849=CARTESIAN_POINT('Origin',(0.,-26.,0.));
#5850=CARTESIAN_POINT('',(-15.,-20.,-1.83697019872103E-15));
#5851=CARTESIAN_POINT('',(-15.,-20.,-1.83697019872103E-15));
#5852=CARTESIAN_POINT('Origin',(0.,-20.,0.));
#5853=CARTESIAN_POINT('Origin',(0.,-26.,0.));
#5854=CARTESIAN_POINT('',(-12.,-26.,-1.46957615897682E-15));
#5855=CARTESIAN_POINT('Origin',(0.,-26.,0.));
#5856=CARTESIAN_POINT('Origin',(0.,-20.,0.));
#5857=CARTESIAN_POINT('',(-12.,-20.,1.46957615897682E-15));
#5858=CARTESIAN_POINT('Origin',(0.,-20.,0.));
#5859=CARTESIAN_POINT('Origin',(0.,20.,0.));
#42647=UNCERTAINTY_MEASURE_WITH_UNIT(LENGTH_MEASURE(0.01),#42668,
'DISTANCE_ACCURACY_VALUE',
'Maximum model space distance between geometric entities at asserted c
onnectivities');
#42656=UNCERTAINTY_MEASURE_WITH_UNIT(LENGTH_MEASURE(0.01),#42668,
'DISTANCE_ACCURACY_VALUE',
'Maximum model space distance between geometric entities at asserted c
onnectivities');
#42658=(
GEOMETRIC_REPRESENTATION_CONTEXT(3)
GLOBAL_UNCERTAINTY_ASSIGNED_CONTEXT((#42647))
GLOBAL_UNIT_ASSIGNED_CONTEXT((#42668,#42670,#42671))
REPRESENTATION_CONTEXT('','3D')
);
#42667=(
GEOMETRIC_REPRESENTATION_CONTEXT(3)
GLOBAL_UNCERTAINTY_ASSIGNED_CONTEXT((#42656))
GLOBAL_UNIT_ASSIGNED_CONTEXT((#42668,#42670,#42671))
REPRESENTATION_CONTEXT('','3D')
);
#42668=(
LENGTH_UNIT()
NAMED_UNIT(*)
SI_UNIT(.MILLI.,.METRE.)
);
#42670=(
NAMED_UNIT(*)
PLANE_ANGLE_UNIT()
SI_UNIT($,.RADIAN.)
);
#42671=(
NAMED_UNIT(*)
SI_UNIT($,.STERADIAN.)
SOLID_ANGLE_UNIT()
);
#42673=SHAPE_DEFINITION_REPRESENTATION(#42683,#42702);
#42683=PRODUCT_DEFINITION_SHAPE('',$,#42713);
#42702=SHAPE_REPRESENTATION('',(#4142),#42658);
#42711=PRODUCT_DEFINITION_CONTEXT('part definition',#42743,'design');
#42713=PRODUCT_DEFINITION('Middle_Body','Middle_Body',#42723,#42711);
#42723=PRODUCT_DEFINITION_FORMATION('',$,#42746);
#42743=APPLICATION_CONTEXT(
'Core Data for Automotive Mechanical Design Process');
#42744=PRODUCT_CONTEXT('part definition',#42743,'mechanical');
#42746=PRODUCT('Middle_Body','Middle_Body',$,(#42744));
#42756=PRESENTATION_STYLE_ASSIGNMENT((#42758));
#42758=SURFACE_STYLE_USAGE(.BOTH.,#42760);
#42760=SURFACE_SIDE_STYLE('',(#42762));
#42762=SURFACE_STYLE_FILL_AREA(#42764);
#42764=FILL_AREA_STYLE('Opaque(160,160,160)',(#42766));
#42766=FILL_AREA_STYLE_COLOUR('Opaque(160,160,160)',#42768);
#42768=COLOUR_RGB('Opaque(160,160,160)', 0.09019608, 0.27058824, 0.51372549);
ENDSEC;
END-ISO-10303-21;
